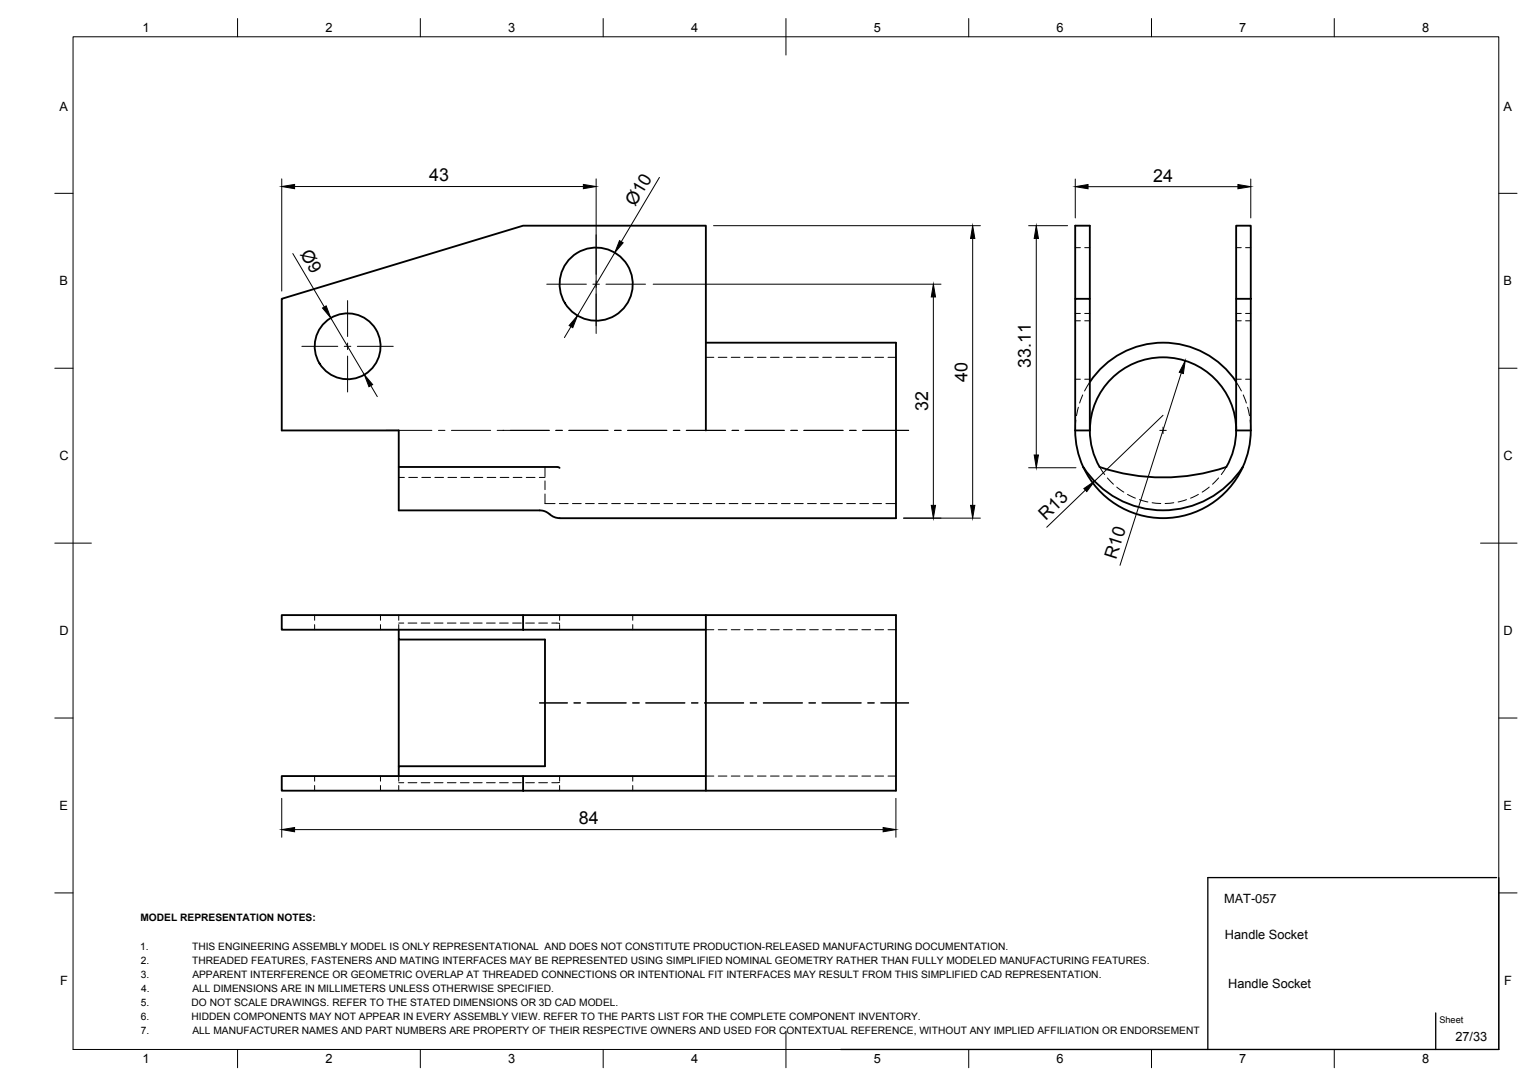
ISO-10303-21;
HEADER;
/* Generated by software containing ST-Developer
 * from STEP Tools, Inc. (www.steptools.com) 
 */

FILE_DESCRIPTION(
/* description */ ('STEP AP214', 'CAx-IF Rec.Pracs.---Representation and Presentation of Product Manufa
cturing Information (PMI)---4.0---2014-10-13'),
/* implementation_level */ '2;1');

FILE_NAME(
/* name */ 'Handle Socket.step',
/* time_stamp */ '2026-10-28T23:34:22+01:00',
/* author */ (''),
/* organization */ (''),
/* preprocessor_version */ 'ST-DEVELOPER v20.2',
/* originating_system */ 'Autodesk Translation Framework v15.17.0.0',
/* authorisation */ '');

FILE_SCHEMA (('AP242_MANAGED_MODEL_BASED_3D_ENGINEERING_MIM_LF { 1 0 10303 442 2 1 4 }'));
ENDSEC;

DATA;
#10=MECHANICAL_DESIGN_GEOMETRIC_PRESENTATION_REPRESENTATION('',(#268),#27807);
#220=SHAPE_REPRESENTATION_RELATIONSHIP('SRR','None',#27918,#242);
#242=ADVANCED_BREP_SHAPE_REPRESENTATION('',(#297),#27798);
#268=STYLED_ITEM('',(#28070),#297);
#297=MANIFOLD_SOLID_BREP('Body1',#12044);
#322=(
BOUNDED_SURFACE()
B_SPLINE_SURFACE(3,2,((#23001,#23002,#23003),(#23004,#23005,#23006),(#23007,
#23008,#23009),(#23010,#23011,#23012),(#23013,#23014,#23015),(#23016,#23017,
#23018),(#23019,#23020,#23021),(#23022,#23023,#23024),(#23025,#23026,#23027),
(#23028,#23029,#23030),(#23031,#23032,#23033),(#23034,#23035,#23036),(#23037,
#23038,#23039),(#23040,#23041,#23042),(#23043,#23044,#23045),(#23046,#23047,
#23048),(#23049,#23050,#23051),(#23052,#23053,#23054),(#23055,#23056,#23057),
(#23058,#23059,#23060),(#23061,#23062,#23063),(#23064,#23065,#23066),(#23067,
#23068,#23069),(#23070,#23071,#23072),(#23073,#23074,#23075),(#23076,#23077,
#23078),(#23079,#23080,#23081),(#23082,#23083,#23084),(#23085,#23086,#23087),
(#23088,#23089,#23090),(#23091,#23092,#23093),(#23094,#23095,#23096),(#23097,
#23098,#23099),(#23100,#23101,#23102),(#23103,#23104,#23105),(#23106,#23107,
#23108),(#23109,#23110,#23111),(#23112,#23113,#23114),(#23115,#23116,#23117),
(#23118,#23119,#23120),(#23121,#23122,#23123),(#23124,#23125,#23126),(#23127,
#23128,#23129),(#23130,#23131,#23132),(#23133,#23134,#23135),(#23136,#23137,
#23138),(#23139,#23140,#23141),(#23142,#23143,#23144),(#23145,#23146,#23147),
(#23148,#23149,#23150),(#23151,#23152,#23153),(#23154,#23155,#23156),(#23157,
#23158,#23159),(#23160,#23161,#23162)),.UNSPECIFIED.,.F.,.F.,.F.)
B_SPLINE_SURFACE_WITH_KNOTS((4,2,2,2,2,2,2,2,2,2,2,2,2,2,2,2,2,2,2,2,2,
2,2,2,2,2,4),(3,3),(0.0156830691858876,0.0164505202472942,0.0166981564596516,
0.0171934288843663,0.017688701309081,0.0181839737337957,0.0191745185832252,
0.0201650634326547,0.0221461531315136,0.0241272428303725,0.025117787679802,
0.0261083325292314,0.0280894222280904,0.0300705119269493,0.0320516016258082,
0.0360137810235261,0.037994870722385,0.0399759604212439,0.0419570501201028,
0.0439381398189618,0.0449286846683912,0.0459192295178207,0.0464145019425354,
0.0469097743672502,0.0474050467919649,0.0476526830043223,0.0484205987519554),
(-0.000176656774630185,1.00140559977643),.UNSPECIFIED.)
GEOMETRIC_REPRESENTATION_ITEM()
RATIONAL_B_SPLINE_SURFACE(((1.00000185229478,0.994749992386749,1.00001475620861),
(1.00000110311236,0.996873419742612,1.0000087878864),(1.00000061689249,
0.998251525466236,1.00000491444144),(1.00000073022143,0.99793031426867,
1.0000058172705),(1.00000081643938,0.997685944476427,1.00000650412124),
(1.00000116817153,0.996689020835744,1.00000930617684),(1.00000151293943,
0.995711836146633,1.00001205275212),(1.00000222875737,0.99368297460525,
1.00001775527797),(1.00000261226297,0.992595994639531,1.00002081045509),
(1.00000339798395,0.990369005078046,1.00002706985983),(1.00000379540439,
0.989242585902711,1.00003023588883),(1.00000499052043,0.985855237206275,
1.00003975671769),(1.00000579086045,0.983586812540499,1.00004613258417),
(1.00000737677408,0.97909181598218,1.00005876668146),(1.00000816422513,
0.976859922850868,1.00006503986867),(1.00001048220609,0.970290008684874,
1.0000835059417),(1.0000119461136,0.966140817279626,1.00009516808364),(1.00001468654717,
0.958373534637283,1.00011699960303),(1.00001596349836,0.954754238433,1.00012717236729),
(1.00001771880672,0.949779121960846,1.00014115593873),(1.00001827868632,
0.948192240535891,1.00014561619005),(1.00001932722233,0.945220347466773,
1.00015396929681),(1.00001981740926,0.943830997788028,1.00015787434518),
(1.00002118448659,0.939956254724288,1.00016876509453),(1.00002195823644,
0.937763195243397,1.00017492913191),(1.00002321565211,0.934199269074837,
1.00018494626748),(1.00002370061483,0.932824726524174,1.00018880969743),
(1.00002434501334,0.930998290964812,1.00019394326411),(1.00002450689124,
0.930539476192181,1.00019523285585),(1.00002450200607,0.930553322329606,
1.00019519393848),(1.00002385083742,0.932398946709429,1.00019000643775),
(1.00002196617021,0.937740708359039,1.00017499233585),(1.00002117811911,
0.939974302221974,1.00016871436838),(1.00001935011025,0.945155475621783,
1.00015415163226),(1.00001830824342,0.948108466066406,1.00014585165514),
(1.00001599049957,0.954677708176843,1.00012738747106),(1.0000147145338,
0.958294211383293,1.00011722255709),(1.00001194082592,0.966155804298885,
1.00009512595959),(1.00001046725737,0.97033237824493,1.00008338685348),
(1.00000815970583,0.976872732002048,1.00006500386596),(1.00000737308074,
0.979102284123733,1.00005873725863),(1.00000577774524,0.983623985306201,
1.0000460281026),(1.00000497387877,0.985902405097253,1.00003962414279),
(1.000003776533,0.989296073600137,1.00003008555083),(1.00000337746495,0.990427162612735,
1.00002690639631),(1.00000259754195,0.992637718792777,1.00002069318092),
(1.00000221666145,0.993717258376601,1.0000176589165),(1.00000150078254,
0.995746292719822,1.00001195590495),(1.00000115795301,0.996717983459339,
1.00000922477153),(1.00000081463085,0.997691070447167,1.00000648971367),
(1.00000072988353,0.997931272000135,1.0000058145786),(1.00000061781061,
0.99824892319208,1.00000492175566),(1.00000109047742,0.996909231281611,
1.00000868723083),(1.00000189977857,0.994615407843422,1.0000151344857)))
REPRESENTATION_ITEM('')
SURFACE()
);
#416=FACE_BOUND('',#2542,.T.);
#417=FACE_BOUND('',#2548,.T.);
#418=FACE_BOUND('',#2549,.T.);
#419=FACE_BOUND('',#2551,.T.);
#420=FACE_BOUND('',#2552,.T.);
#421=FACE_BOUND('',#2558,.T.);
#422=FACE_BOUND('',#2559,.T.);
#423=FACE_BOUND('',#2561,.T.);
#424=FACE_BOUND('',#2562,.T.);
#671=PLANE('',#13398);
#672=PLANE('',#13399);
#673=PLANE('',#13400);
#674=PLANE('',#13401);
#675=PLANE('',#13402);
#676=PLANE('',#13403);
#677=PLANE('',#13404);
#678=PLANE('',#13405);
#679=PLANE('',#13406);
#680=PLANE('',#13407);
#681=PLANE('',#13408);
#682=PLANE('',#13409);
#683=PLANE('',#13410);
#684=PLANE('',#13411);
#685=PLANE('',#13412);
#686=PLANE('',#13413);
#687=PLANE('',#13419);
#688=PLANE('',#13420);
#838=TOROIDAL_SURFACE('',#13421,10.,2.);
#920=B_SPLINE_CURVE_WITH_KNOTS('',3,(#22599,#22600,#22601,#22602,#22603,
#22604,#22605,#22606,#22607,#22608,#22609,#22610,#22611),.UNSPECIFIED.,
 .F.,.F.,(4,3,3,3,4),(-8.94491631300586E-6,0.000122293976412443,0.000196963243301103,
0.000348477111734026,0.000402871401407367),.UNSPECIFIED.);
#921=B_SPLINE_CURVE_WITH_KNOTS('',3,(#22635,#22636,#22637,#22638,#22639,
#22640,#22641,#22642,#22643,#22644,#22645,#22646,#22647),.UNSPECIFIED.,
 .F.,.F.,(4,3,3,3,4),(1.90501246655379E-12,0.000149886598358764,0.000203002185902805,
0.000344863019354018,0.000406004371347535),.UNSPECIFIED.);
#922=B_SPLINE_CURVE_WITH_KNOTS('',3,(#22716,#22717,#22718,#22719,#22720,
#22721,#22722,#22723,#22724,#22725,#22726,#22727,#22728,#22729,#22730,#22731,
#22732,#22733,#22734,#22735,#22736,#22737,#22738,#22739,#22740,#22741,#22742,
#22743,#22744,#22745,#22746,#22747,#22748,#22749,#22750,#22751,#22752,#22753,
#22754,#22755,#22756,#22757,#22758,#22759,#22760,#22761),.UNSPECIFIED.,
 .F.,.F.,(4,2,2,2,2,2,2,2,2,2,2,2,2,2,2,2,2,2,2,2,2,2,4),(0.,0.00042797836355374,
0.00085595672710748,0.00171191345421505,0.00256787018132261,0.00342382690843018,
0.00513574036264529,0.00684765381686041,0.00770361054396788,0.00855956727107535,
0.0102714807252903,0.0119833941795052,0.0136953076337201,0.0171191345421499,
0.0188310479963648,0.0205429614505798,0.0222548749047947,0.0239667883590096,
0.0248227450861171,0.0256787018132246,0.0265346585403321,0.0269626369038859,
0.0273906152674397),.UNSPECIFIED.);
#923=B_SPLINE_CURVE_WITH_KNOTS('',3,(#22766,#22767,#22768,#22769,#22770,
#22771,#22772,#22773,#22774,#22775,#22776,#22777,#22778,#22779,#22780,#22781,
#22782,#22783,#22784,#22785,#22786,#22787,#22788,#22789,#22790,#22791,#22792,
#22793,#22794,#22795,#22796,#22797,#22798,#22799,#22800,#22801,#22802,#22803,
#22804,#22805,#22806,#22807,#22808,#22809,#22810,#22811,#22812,#22813,#22814,
#22815,#22816,#22817,#22818,#22819,#22820,#22821,#22822,#22823,#22824,#22825,
#22826,#22827,#22828,#22829,#22830,#22831,#22832,#22833,#22834,#22835,#22836,
#22837,#22838,#22839,#22840,#22841,#22842,#22843,#22844,#22845,#22846,#22847,
#22848,#22849,#22850,#22851,#22852,#22853,#22854,#22855,#22856,#22857,#22858,
#22859,#22860,#22861,#22862,#22863,#22864,#22865,#22866,#22867,#22868,#22869,
#22870,#22871,#22872,#22873,#22874,#22875,#22876,#22877,#22878,#22879,#22880,
#22881,#22882,#22883,#22884,#22885,#22886,#22887,#22888,#22889,#22890,#22891,
#22892,#22893,#22894,#22895,#22896,#22897,#22898,#22899,#22900,#22901,#22902,
#22903,#22904,#22905,#22906,#22907,#22908,#22909,#22910,#22911,#22912,#22913,
#22914,#22915,#22916,#22917,#22918,#22919,#22920,#22921,#22922,#22923,#22924,
#22925,#22926,#22927,#22928,#22929,#22930,#22931,#22932,#22933,#22934,#22935,
#22936,#22937,#22938,#22939,#22940,#22941,#22942,#22943,#22944,#22945,#22946,
#22947,#22948,#22949,#22950,#22951,#22952,#22953,#22954,#22955,#22956,#22957,
#22958,#22959,#22960,#22961,#22962,#22963,#22964,#22965,#22966,#22967,#22968,
#22969,#22970,#22971,#22972,#22973,#22974,#22975,#22976,#22977,#22978,#22979,
#22980,#22981,#22982,#22983,#22984,#22985,#22986,#22987,#22988,#22989,#22990,
#22991,#22992,#22993,#22994,#22995,#22996,#22997,#22998,#22999,#23000),
 .UNSPECIFIED.,.F.,.F.,(4,3,3,3,3,3,3,3,3,3,3,3,3,3,3,3,3,3,3,3,3,3,3,3,
3,3,3,3,3,3,3,3,3,3,3,3,3,3,3,3,3,3,3,3,3,3,3,3,3,3,3,3,3,3,3,3,3,3,3,3,
3,3,3,3,3,3,3,3,3,3,3,3,3,3,3,3,3,3,4),(4.92899567643811E-13,6.25324094450888E-5,
0.000108135161089233,0.000169914174680728,0.000216270322178465,0.00030943720716885,
0.000413935938866143,0.000432540644356983,0.000574368182756462,0.000730585733412546,
0.000865081288713848,0.0011111676997501,0.00137115397560176,0.00165280502519303,
0.00173016257742746,0.0021631859889676,0.00262174667632143,0.00312444156864647,
0.00346032515485454,0.00399962729951328,0.00432540644356815,0.00475794708792495,
0.00519048773228175,0.00580087629302463,0.0064255985829778,0.00692065030970915,
0.00756964026772925,0.00822018102493731,0.00865081288713655,0.00908335353149343,
0.00949422462642801,0.00951589417585031,0.0101632105932538,0.0103809754645641,
0.0110451277363797,0.0117441709571396,0.0124097069791447,0.0130727965065704,
0.0137303575905069,0.0138413006194192,0.0145176167184007,0.0151956374788783,
0.0155714631968468,0.0160965814245652,0.0166216819946583,0.0171475979342611,
0.0173016257742743,0.0179650597324343,0.018627559129564,0.0190317883517019,
0.0198298746356556,0.0206344291379891,0.0207619509291294,0.0213868246193969,
0.022007159801814,0.022492113506557,0.0230625131047404,0.0236423945943625,
0.0241817119047142,0.0242222760839846,0.0246853332276435,0.0250873573726984,
0.0254771261541672,0.025844738861123,0.0259524386614121,0.0262218968916945,
0.0264777260220052,0.0267146153189825,0.0268175199501259,0.0269752262516356,
0.0271182846351551,0.0272500605944827,0.0273581957555719,0.0274515657429817,
0.0274663309166611,0.0275422189045734,0.0275744660777502,0.027633797106646,
0.0276826012383845),.UNSPECIFIED.);
#1167=CYLINDRICAL_SURFACE('',#13370,4.50000000000001);
#1168=CYLINDRICAL_SURFACE('',#13373,4.99999999999999);
#1169=CYLINDRICAL_SURFACE('',#13376,4.50000000000001);
#1170=CYLINDRICAL_SURFACE('',#13379,4.99999999999999);
#1171=CYLINDRICAL_SURFACE('',#13382,10.);
#1172=CYLINDRICAL_SURFACE('',#13389,12.);
#1173=CYLINDRICAL_SURFACE('',#13414,27.);
#1174=CYLINDRICAL_SURFACE('',#13417,13.);
#1754=FACE_OUTER_BOUND('',#2532,.T.);
#1755=FACE_OUTER_BOUND('',#2533,.T.);
#1756=FACE_OUTER_BOUND('',#2534,.T.);
#1757=FACE_OUTER_BOUND('',#2535,.T.);
#1758=FACE_OUTER_BOUND('',#2536,.T.);
#1759=FACE_OUTER_BOUND('',#2537,.T.);
#1760=FACE_OUTER_BOUND('',#2538,.T.);
#1761=FACE_OUTER_BOUND('',#2539,.T.);
#1762=FACE_OUTER_BOUND('',#2540,.T.);
#1763=FACE_OUTER_BOUND('',#2541,.T.);
#1764=FACE_OUTER_BOUND('',#2543,.T.);
#1765=FACE_OUTER_BOUND('',#2544,.T.);
#1766=FACE_OUTER_BOUND('',#2545,.T.);
#1767=FACE_OUTER_BOUND('',#2546,.T.);
#1768=FACE_OUTER_BOUND('',#2547,.T.);
#1769=FACE_OUTER_BOUND('',#2550,.T.);
#1770=FACE_OUTER_BOUND('',#2553,.T.);
#1771=FACE_OUTER_BOUND('',#2554,.T.);
#1772=FACE_OUTER_BOUND('',#2555,.T.);
#1773=FACE_OUTER_BOUND('',#2556,.T.);
#1774=FACE_OUTER_BOUND('',#2557,.T.);
#1775=FACE_OUTER_BOUND('',#2560,.T.);
#1776=FACE_OUTER_BOUND('',#2563,.T.);
#1777=FACE_OUTER_BOUND('',#2564,.T.);
#1778=FACE_OUTER_BOUND('',#2565,.T.);
#1779=FACE_OUTER_BOUND('',#2566,.T.);
#1780=FACE_OUTER_BOUND('',#2567,.T.);
#1781=FACE_OUTER_BOUND('',#2568,.T.);
#2532=EDGE_LOOP('',(#10371,#10372,#10373,#10374));
#2533=EDGE_LOOP('',(#10375,#10376,#10377,#10378));
#2534=EDGE_LOOP('',(#10379,#10380,#10381,#10382));
#2535=EDGE_LOOP('',(#10383,#10384,#10385,#10386));
#2536=EDGE_LOOP('',(#10387,#10388,#10389,#10390,#10391,#10392,#10393,#10394,
#10395,#10396,#10397,#10398));
#2537=EDGE_LOOP('',(#10399,#10400,#10401,#10402,#10403,#10404,#10405,#10406,
#10407,#10408,#10409,#10410,#10411,#10412,#10413,#10414));
#2538=EDGE_LOOP('',(#10415,#10416,#10417,#10418));
#2539=EDGE_LOOP('',(#10419,#10420,#10421,#10422));
#2540=EDGE_LOOP('',(#10423,#10424,#10425,#10426,#10427,#10428));
#2541=EDGE_LOOP('',(#10429));
#2542=EDGE_LOOP('',(#10430));
#2543=EDGE_LOOP('',(#10431,#10432,#10433,#10434));
#2544=EDGE_LOOP('',(#10435,#10436,#10437,#10438));
#2545=EDGE_LOOP('',(#10439,#10440,#10441,#10442));
#2546=EDGE_LOOP('',(#10443,#10444,#10445,#10446));
#2547=EDGE_LOOP('',(#10447,#10448,#10449,#10450,#10451,#10452));
#2548=EDGE_LOOP('',(#10453));
#2549=EDGE_LOOP('',(#10454));
#2550=EDGE_LOOP('',(#10455,#10456,#10457,#10458,#10459,#10460,#10461));
#2551=EDGE_LOOP('',(#10462));
#2552=EDGE_LOOP('',(#10463));
#2553=EDGE_LOOP('',(#10464,#10465,#10466,#10467));
#2554=EDGE_LOOP('',(#10468,#10469,#10470,#10471));
#2555=EDGE_LOOP('',(#10472,#10473,#10474,#10475));
#2556=EDGE_LOOP('',(#10476,#10477,#10478,#10479));
#2557=EDGE_LOOP('',(#10480,#10481,#10482,#10483,#10484,#10485));
#2558=EDGE_LOOP('',(#10486));
#2559=EDGE_LOOP('',(#10487));
#2560=EDGE_LOOP('',(#10488,#10489,#10490,#10491,#10492,#10493,#10494));
#2561=EDGE_LOOP('',(#10495));
#2562=EDGE_LOOP('',(#10496));
#2563=EDGE_LOOP('',(#10497,#10498,#10499,#10500));
#2564=EDGE_LOOP('',(#10501,#10502,#10503,#10504));
#2565=EDGE_LOOP('',(#10505,#10506,#10507,#10508,#10509,#10510,#10511,#10512));
#2566=EDGE_LOOP('',(#10513,#10514));
#2567=EDGE_LOOP('',(#10515,#10516));
#2568=EDGE_LOOP('',(#10517,#10518,#10519,#10520));
#3372=LINE('',#22552,#4192);
#3373=LINE('',#22558,#4193);
#3374=LINE('',#22564,#4194);
#3375=LINE('',#22570,#4195);
#3376=LINE('',#22576,#4196);
#3377=LINE('',#22580,#4197);
#3378=LINE('',#22584,#4198);
#3379=LINE('',#22588,#4199);
#3380=LINE('',#22592,#4200);
#3381=LINE('',#22613,#4201);
#3382=LINE('',#22617,#4202);
#3383=LINE('',#22623,#4203);
#3384=LINE('',#22630,#4204);
#3385=LINE('',#22634,#4205);
#3386=LINE('',#22650,#4206);
#3387=LINE('',#22651,#4207);
#3388=LINE('',#22653,#4208);
#3389=LINE('',#22654,#4209);
#3390=LINE('',#22656,#4210);
#3391=LINE('',#22658,#4211);
#3392=LINE('',#22660,#4212);
#3393=LINE('',#22661,#4213);
#3394=LINE('',#22663,#4214);
#3395=LINE('',#22664,#4215);
#3396=LINE('',#22668,#4216);
#3397=LINE('',#22670,#4217);
#3398=LINE('',#22671,#4218);
#3399=LINE('',#22674,#4219);
#3400=LINE('',#22676,#4220);
#3401=LINE('',#22677,#4221);
#3402=LINE('',#22680,#4222);
#3403=LINE('',#22682,#4223);
#3404=LINE('',#22683,#4224);
#3405=LINE('',#22685,#4225);
#3406=LINE('',#22686,#4226);
#3407=LINE('',#22691,#4227);
#3408=LINE('',#22693,#4228);
#3409=LINE('',#22694,#4229);
#3410=LINE('',#22697,#4230);
#3411=LINE('',#22699,#4231);
#3412=LINE('',#22700,#4232);
#3413=LINE('',#22703,#4233);
#3414=LINE('',#22705,#4234);
#3415=LINE('',#22706,#4235);
#3416=LINE('',#22708,#4236);
#3417=LINE('',#22709,#4237);
#4192=VECTOR('',#16498,4.50000000000001);
#4193=VECTOR('',#16505,4.99999999999999);
#4194=VECTOR('',#16512,4.50000000000001);
#4195=VECTOR('',#16519,4.99999999999999);
#4196=VECTOR('',#16526,10.);
#4197=VECTOR('',#16529,1000.);
#4198=VECTOR('',#16532,1000.);
#4199=VECTOR('',#16535,1000.);
#4200=VECTOR('',#16538,1000.);
#4201=VECTOR('',#16545,1000.);
#4202=VECTOR('',#16548,1000.);
#4203=VECTOR('',#16553,12.);
#4204=VECTOR('',#16560,1000.);
#4205=VECTOR('',#16563,1000.);
#4206=VECTOR('',#16566,1000.);
#4207=VECTOR('',#16567,1000.);
#4208=VECTOR('',#16568,1000.);
#4209=VECTOR('',#16569,1000.);
#4210=VECTOR('',#16572,1000.);
#4211=VECTOR('',#16573,1000.);
#4212=VECTOR('',#16574,1000.);
#4213=VECTOR('',#16575,1000.);
#4214=VECTOR('',#16578,1000.);
#4215=VECTOR('',#16579,1000.);
#4216=VECTOR('',#16584,1000.);
#4217=VECTOR('',#16585,1000.);
#4218=VECTOR('',#16586,1000.);
#4219=VECTOR('',#16589,1000.);
#4220=VECTOR('',#16590,1000.);
#4221=VECTOR('',#16591,1000.);
#4222=VECTOR('',#16594,1000.);
#4223=VECTOR('',#16595,1000.);
#4224=VECTOR('',#16596,1000.);
#4225=VECTOR('',#16599,1000.);
#4226=VECTOR('',#16600,1000.);
#4227=VECTOR('',#16607,1000.);
#4228=VECTOR('',#16608,1000.);
#4229=VECTOR('',#16609,1000.);
#4230=VECTOR('',#16612,1000.);
#4231=VECTOR('',#16613,1000.);
#4232=VECTOR('',#16614,1000.);
#4233=VECTOR('',#16617,1000.);
#4234=VECTOR('',#16618,1000.);
#4235=VECTOR('',#16619,1000.);
#4236=VECTOR('',#16622,1000.);
#4237=VECTOR('',#16623,1000.);
#4893=CIRCLE('',#13371,4.50000000000001);
#4894=CIRCLE('',#13372,4.50000000000001);
#4895=CIRCLE('',#13374,4.99999999999999);
#4896=CIRCLE('',#13375,4.99999999999999);
#4897=CIRCLE('',#13377,4.50000000000001);
#4898=CIRCLE('',#13378,4.50000000000001);
#4899=CIRCLE('',#13380,4.99999999999999);
#4900=CIRCLE('',#13381,4.99999999999999);
#4901=CIRCLE('',#13383,10.);
#4902=CIRCLE('',#13384,10.);
#4903=CIRCLE('',#13385,10.);
#4904=CIRCLE('',#13386,10.);
#4905=CIRCLE('',#13387,10.);
#4906=CIRCLE('',#13388,10.);
#4907=CIRCLE('',#13390,12.);
#4908=CIRCLE('',#13391,12.);
#4909=CIRCLE('',#13392,12.);
#4910=CIRCLE('',#13393,12.);
#4911=CIRCLE('',#13394,12.);
#4912=CIRCLE('',#13395,12.);
#4913=CIRCLE('',#13396,12.);
#4914=CIRCLE('',#13397,12.);
#4915=CIRCLE('',#13415,27.);
#4916=CIRCLE('',#13416,27.);
#4917=CIRCLE('',#13418,13.);
#5843=VERTEX_POINT('',#22549);
#5844=VERTEX_POINT('',#22551);
#5845=VERTEX_POINT('',#22555);
#5846=VERTEX_POINT('',#22557);
#5847=VERTEX_POINT('',#22561);
#5848=VERTEX_POINT('',#22563);
#5849=VERTEX_POINT('',#22567);
#5850=VERTEX_POINT('',#22569);
#5851=VERTEX_POINT('',#22573);
#5852=VERTEX_POINT('',#22575);
#5853=VERTEX_POINT('',#22577);
#5854=VERTEX_POINT('',#22579);
#5855=VERTEX_POINT('',#22581);
#5856=VERTEX_POINT('',#22583);
#5857=VERTEX_POINT('',#22585);
#5858=VERTEX_POINT('',#22587);
#5859=VERTEX_POINT('',#22589);
#5860=VERTEX_POINT('',#22591);
#5861=VERTEX_POINT('',#22595);
#5862=VERTEX_POINT('',#22596);
#5863=VERTEX_POINT('',#22598);
#5864=VERTEX_POINT('',#22612);
#5865=VERTEX_POINT('',#22614);
#5866=VERTEX_POINT('',#22616);
#5867=VERTEX_POINT('',#22618);
#5868=VERTEX_POINT('',#22620);
#5869=VERTEX_POINT('',#22622);
#5870=VERTEX_POINT('',#22625);
#5871=VERTEX_POINT('',#22627);
#5872=VERTEX_POINT('',#22629);
#5873=VERTEX_POINT('',#22631);
#5874=VERTEX_POINT('',#22633);
#5875=VERTEX_POINT('',#22649);
#5876=VERTEX_POINT('',#22652);
#5877=VERTEX_POINT('',#22657);
#5878=VERTEX_POINT('',#22659);
#5879=VERTEX_POINT('',#22667);
#5880=VERTEX_POINT('',#22669);
#5881=VERTEX_POINT('',#22673);
#5882=VERTEX_POINT('',#22675);
#5883=VERTEX_POINT('',#22679);
#5884=VERTEX_POINT('',#22681);
#5885=VERTEX_POINT('',#22690);
#5886=VERTEX_POINT('',#22692);
#5887=VERTEX_POINT('',#22696);
#5888=VERTEX_POINT('',#22698);
#5889=VERTEX_POINT('',#22702);
#5890=VERTEX_POINT('',#22704);
#7398=EDGE_CURVE('',#5843,#5843,#4893,.T.);
#7399=EDGE_CURVE('',#5843,#5844,#3372,.T.);
#7400=EDGE_CURVE('',#5844,#5844,#4894,.T.);
#7401=EDGE_CURVE('',#5845,#5845,#4895,.T.);
#7402=EDGE_CURVE('',#5845,#5846,#3373,.T.);
#7403=EDGE_CURVE('',#5846,#5846,#4896,.T.);
#7404=EDGE_CURVE('',#5847,#5847,#4897,.T.);
#7405=EDGE_CURVE('',#5847,#5848,#3374,.T.);
#7406=EDGE_CURVE('',#5848,#5848,#4898,.T.);
#7407=EDGE_CURVE('',#5849,#5849,#4899,.T.);
#7408=EDGE_CURVE('',#5849,#5850,#3375,.T.);
#7409=EDGE_CURVE('',#5850,#5850,#4900,.T.);
#7410=EDGE_CURVE('',#5851,#5851,#4901,.T.);
#7411=EDGE_CURVE('',#5851,#5852,#3376,.T.);
#7412=EDGE_CURVE('',#5852,#5853,#4902,.T.);
#7413=EDGE_CURVE('',#5854,#5853,#3377,.T.);
#7414=EDGE_CURVE('',#5855,#5854,#4903,.T.);
#7415=EDGE_CURVE('',#5855,#5856,#3378,.T.);
#7416=EDGE_CURVE('',#5857,#5856,#4904,.T.);
#7417=EDGE_CURVE('',#5858,#5857,#3379,.T.);
#7418=EDGE_CURVE('',#5859,#5858,#4905,.T.);
#7419=EDGE_CURVE('',#5860,#5859,#3380,.T.);
#7420=EDGE_CURVE('',#5860,#5852,#4906,.T.);
#7421=EDGE_CURVE('',#5861,#5862,#4907,.T.);
#7422=EDGE_CURVE('',#5862,#5863,#920,.T.);
#7423=EDGE_CURVE('',#5864,#5863,#3381,.T.);
#7424=EDGE_CURVE('',#5865,#5864,#4908,.T.);
#7425=EDGE_CURVE('',#5865,#5866,#3382,.T.);
#7426=EDGE_CURVE('',#5866,#5867,#4909,.T.);
#7427=EDGE_CURVE('',#5868,#5867,#4910,.T.);
#7428=EDGE_CURVE('',#5868,#5869,#3383,.T.);
#7429=EDGE_CURVE('',#5869,#5869,#4911,.T.);
#7430=EDGE_CURVE('',#5870,#5868,#4912,.T.);
#7431=EDGE_CURVE('',#5871,#5870,#4913,.T.);
#7432=EDGE_CURVE('',#5871,#5872,#3384,.T.);
#7433=EDGE_CURVE('',#5873,#5872,#4914,.T.);
#7434=EDGE_CURVE('',#5873,#5874,#3385,.T.);
#7435=EDGE_CURVE('',#5874,#5861,#921,.T.);
#7436=EDGE_CURVE('',#5859,#5875,#3386,.T.);
#7437=EDGE_CURVE('',#5872,#5859,#3387,.T.);
#7438=EDGE_CURVE('',#5872,#5876,#3388,.T.);
#7439=EDGE_CURVE('',#5876,#5875,#3389,.T.);
#7440=EDGE_CURVE('',#5854,#5865,#3390,.T.);
#7441=EDGE_CURVE('',#5854,#5877,#3391,.T.);
#7442=EDGE_CURVE('',#5878,#5877,#3392,.T.);
#7443=EDGE_CURVE('',#5865,#5878,#3393,.T.);
#7444=EDGE_CURVE('',#5853,#5867,#3394,.T.);
#7445=EDGE_CURVE('',#5860,#5870,#3395,.T.);
#7446=EDGE_CURVE('',#5871,#5879,#3396,.T.);
#7447=EDGE_CURVE('',#5870,#5880,#3397,.T.);
#7448=EDGE_CURVE('',#5879,#5880,#3398,.T.);
#7449=EDGE_CURVE('',#5880,#5881,#3399,.T.);
#7450=EDGE_CURVE('',#5882,#5881,#3400,.T.);
#7451=EDGE_CURVE('',#5879,#5882,#3401,.T.);
#7452=EDGE_CURVE('',#5881,#5883,#3402,.T.);
#7453=EDGE_CURVE('',#5884,#5883,#3403,.T.);
#7454=EDGE_CURVE('',#5882,#5884,#3404,.T.);
#7455=EDGE_CURVE('',#5875,#5883,#3405,.T.);
#7456=EDGE_CURVE('',#5876,#5884,#3406,.T.);
#7457=EDGE_CURVE('',#5866,#5885,#3407,.T.);
#7458=EDGE_CURVE('',#5885,#5886,#3408,.T.);
#7459=EDGE_CURVE('',#5867,#5886,#3409,.T.);
#7460=EDGE_CURVE('',#5886,#5887,#3410,.T.);
#7461=EDGE_CURVE('',#5885,#5888,#3411,.T.);
#7462=EDGE_CURVE('',#5888,#5887,#3412,.T.);
#7463=EDGE_CURVE('',#5877,#5889,#3413,.T.);
#7464=EDGE_CURVE('',#5890,#5889,#3414,.T.);
#7465=EDGE_CURVE('',#5878,#5890,#3415,.T.);
#7466=EDGE_CURVE('',#5887,#5889,#3416,.T.);
#7467=EDGE_CURVE('',#5888,#5890,#3417,.T.);
#7468=EDGE_CURVE('',#5857,#5856,#4915,.T.);
#7469=EDGE_CURVE('',#5858,#5855,#4916,.T.);
#7470=EDGE_CURVE('',#5863,#5874,#922,.T.);
#7471=EDGE_CURVE('',#5864,#5873,#4917,.T.);
#7472=EDGE_CURVE('',#5861,#5862,#923,.T.);
#10371=ORIENTED_EDGE('',*,*,#7398,.F.);
#10372=ORIENTED_EDGE('',*,*,#7399,.T.);
#10373=ORIENTED_EDGE('',*,*,#7400,.T.);
#10374=ORIENTED_EDGE('',*,*,#7399,.F.);
#10375=ORIENTED_EDGE('',*,*,#7401,.F.);
#10376=ORIENTED_EDGE('',*,*,#7402,.T.);
#10377=ORIENTED_EDGE('',*,*,#7403,.T.);
#10378=ORIENTED_EDGE('',*,*,#7402,.F.);
#10379=ORIENTED_EDGE('',*,*,#7404,.T.);
#10380=ORIENTED_EDGE('',*,*,#7405,.T.);
#10381=ORIENTED_EDGE('',*,*,#7406,.F.);
#10382=ORIENTED_EDGE('',*,*,#7405,.F.);
#10383=ORIENTED_EDGE('',*,*,#7407,.T.);
#10384=ORIENTED_EDGE('',*,*,#7408,.T.);
#10385=ORIENTED_EDGE('',*,*,#7409,.F.);
#10386=ORIENTED_EDGE('',*,*,#7408,.F.);
#10387=ORIENTED_EDGE('',*,*,#7410,.T.);
#10388=ORIENTED_EDGE('',*,*,#7411,.T.);
#10389=ORIENTED_EDGE('',*,*,#7412,.T.);
#10390=ORIENTED_EDGE('',*,*,#7413,.F.);
#10391=ORIENTED_EDGE('',*,*,#7414,.F.);
#10392=ORIENTED_EDGE('',*,*,#7415,.T.);
#10393=ORIENTED_EDGE('',*,*,#7416,.F.);
#10394=ORIENTED_EDGE('',*,*,#7417,.F.);
#10395=ORIENTED_EDGE('',*,*,#7418,.F.);
#10396=ORIENTED_EDGE('',*,*,#7419,.F.);
#10397=ORIENTED_EDGE('',*,*,#7420,.T.);
#10398=ORIENTED_EDGE('',*,*,#7411,.F.);
#10399=ORIENTED_EDGE('',*,*,#7421,.T.);
#10400=ORIENTED_EDGE('',*,*,#7422,.T.);
#10401=ORIENTED_EDGE('',*,*,#7423,.F.);
#10402=ORIENTED_EDGE('',*,*,#7424,.F.);
#10403=ORIENTED_EDGE('',*,*,#7425,.T.);
#10404=ORIENTED_EDGE('',*,*,#7426,.T.);
#10405=ORIENTED_EDGE('',*,*,#7427,.F.);
#10406=ORIENTED_EDGE('',*,*,#7428,.T.);
#10407=ORIENTED_EDGE('',*,*,#7429,.F.);
#10408=ORIENTED_EDGE('',*,*,#7428,.F.);
#10409=ORIENTED_EDGE('',*,*,#7430,.F.);
#10410=ORIENTED_EDGE('',*,*,#7431,.F.);
#10411=ORIENTED_EDGE('',*,*,#7432,.T.);
#10412=ORIENTED_EDGE('',*,*,#7433,.F.);
#10413=ORIENTED_EDGE('',*,*,#7434,.T.);
#10414=ORIENTED_EDGE('',*,*,#7435,.T.);
#10415=ORIENTED_EDGE('',*,*,#7436,.F.);
#10416=ORIENTED_EDGE('',*,*,#7437,.F.);
#10417=ORIENTED_EDGE('',*,*,#7438,.T.);
#10418=ORIENTED_EDGE('',*,*,#7439,.T.);
#10419=ORIENTED_EDGE('',*,*,#7440,.F.);
#10420=ORIENTED_EDGE('',*,*,#7441,.T.);
#10421=ORIENTED_EDGE('',*,*,#7442,.F.);
#10422=ORIENTED_EDGE('',*,*,#7443,.F.);
#10423=ORIENTED_EDGE('',*,*,#7430,.T.);
#10424=ORIENTED_EDGE('',*,*,#7427,.T.);
#10425=ORIENTED_EDGE('',*,*,#7444,.F.);
#10426=ORIENTED_EDGE('',*,*,#7412,.F.);
#10427=ORIENTED_EDGE('',*,*,#7420,.F.);
#10428=ORIENTED_EDGE('',*,*,#7445,.T.);
#10429=ORIENTED_EDGE('',*,*,#7429,.T.);
#10430=ORIENTED_EDGE('',*,*,#7410,.F.);
#10431=ORIENTED_EDGE('',*,*,#7446,.F.);
#10432=ORIENTED_EDGE('',*,*,#7431,.T.);
#10433=ORIENTED_EDGE('',*,*,#7447,.T.);
#10434=ORIENTED_EDGE('',*,*,#7448,.F.);
#10435=ORIENTED_EDGE('',*,*,#7449,.T.);
#10436=ORIENTED_EDGE('',*,*,#7450,.F.);
#10437=ORIENTED_EDGE('',*,*,#7451,.F.);
#10438=ORIENTED_EDGE('',*,*,#7448,.T.);
#10439=ORIENTED_EDGE('',*,*,#7452,.T.);
#10440=ORIENTED_EDGE('',*,*,#7453,.F.);
#10441=ORIENTED_EDGE('',*,*,#7454,.F.);
#10442=ORIENTED_EDGE('',*,*,#7450,.T.);
#10443=ORIENTED_EDGE('',*,*,#7455,.F.);
#10444=ORIENTED_EDGE('',*,*,#7439,.F.);
#10445=ORIENTED_EDGE('',*,*,#7456,.T.);
#10446=ORIENTED_EDGE('',*,*,#7453,.T.);
#10447=ORIENTED_EDGE('',*,*,#7451,.T.);
#10448=ORIENTED_EDGE('',*,*,#7454,.T.);
#10449=ORIENTED_EDGE('',*,*,#7456,.F.);
#10450=ORIENTED_EDGE('',*,*,#7438,.F.);
#10451=ORIENTED_EDGE('',*,*,#7432,.F.);
#10452=ORIENTED_EDGE('',*,*,#7446,.T.);
#10453=ORIENTED_EDGE('',*,*,#7404,.F.);
#10454=ORIENTED_EDGE('',*,*,#7407,.F.);
#10455=ORIENTED_EDGE('',*,*,#7449,.F.);
#10456=ORIENTED_EDGE('',*,*,#7447,.F.);
#10457=ORIENTED_EDGE('',*,*,#7445,.F.);
#10458=ORIENTED_EDGE('',*,*,#7419,.T.);
#10459=ORIENTED_EDGE('',*,*,#7436,.T.);
#10460=ORIENTED_EDGE('',*,*,#7455,.T.);
#10461=ORIENTED_EDGE('',*,*,#7452,.F.);
#10462=ORIENTED_EDGE('',*,*,#7406,.T.);
#10463=ORIENTED_EDGE('',*,*,#7409,.T.);
#10464=ORIENTED_EDGE('',*,*,#7426,.F.);
#10465=ORIENTED_EDGE('',*,*,#7457,.T.);
#10466=ORIENTED_EDGE('',*,*,#7458,.T.);
#10467=ORIENTED_EDGE('',*,*,#7459,.F.);
#10468=ORIENTED_EDGE('',*,*,#7460,.F.);
#10469=ORIENTED_EDGE('',*,*,#7458,.F.);
#10470=ORIENTED_EDGE('',*,*,#7461,.T.);
#10471=ORIENTED_EDGE('',*,*,#7462,.T.);
#10472=ORIENTED_EDGE('',*,*,#7463,.T.);
#10473=ORIENTED_EDGE('',*,*,#7464,.F.);
#10474=ORIENTED_EDGE('',*,*,#7465,.F.);
#10475=ORIENTED_EDGE('',*,*,#7442,.T.);
#10476=ORIENTED_EDGE('',*,*,#7466,.F.);
#10477=ORIENTED_EDGE('',*,*,#7462,.F.);
#10478=ORIENTED_EDGE('',*,*,#7467,.T.);
#10479=ORIENTED_EDGE('',*,*,#7464,.T.);
#10480=ORIENTED_EDGE('',*,*,#7461,.F.);
#10481=ORIENTED_EDGE('',*,*,#7457,.F.);
#10482=ORIENTED_EDGE('',*,*,#7425,.F.);
#10483=ORIENTED_EDGE('',*,*,#7443,.T.);
#10484=ORIENTED_EDGE('',*,*,#7465,.T.);
#10485=ORIENTED_EDGE('',*,*,#7467,.F.);
#10486=ORIENTED_EDGE('',*,*,#7398,.T.);
#10487=ORIENTED_EDGE('',*,*,#7401,.T.);
#10488=ORIENTED_EDGE('',*,*,#7460,.T.);
#10489=ORIENTED_EDGE('',*,*,#7466,.T.);
#10490=ORIENTED_EDGE('',*,*,#7463,.F.);
#10491=ORIENTED_EDGE('',*,*,#7441,.F.);
#10492=ORIENTED_EDGE('',*,*,#7413,.T.);
#10493=ORIENTED_EDGE('',*,*,#7444,.T.);
#10494=ORIENTED_EDGE('',*,*,#7459,.T.);
#10495=ORIENTED_EDGE('',*,*,#7400,.F.);
#10496=ORIENTED_EDGE('',*,*,#7403,.F.);
#10497=ORIENTED_EDGE('',*,*,#7468,.T.);
#10498=ORIENTED_EDGE('',*,*,#7415,.F.);
#10499=ORIENTED_EDGE('',*,*,#7469,.F.);
#10500=ORIENTED_EDGE('',*,*,#7417,.T.);
#10501=ORIENTED_EDGE('',*,*,#7423,.T.);
#10502=ORIENTED_EDGE('',*,*,#7470,.T.);
#10503=ORIENTED_EDGE('',*,*,#7434,.F.);
#10504=ORIENTED_EDGE('',*,*,#7471,.F.);
#10505=ORIENTED_EDGE('',*,*,#7418,.T.);
#10506=ORIENTED_EDGE('',*,*,#7469,.T.);
#10507=ORIENTED_EDGE('',*,*,#7414,.T.);
#10508=ORIENTED_EDGE('',*,*,#7440,.T.);
#10509=ORIENTED_EDGE('',*,*,#7424,.T.);
#10510=ORIENTED_EDGE('',*,*,#7471,.T.);
#10511=ORIENTED_EDGE('',*,*,#7433,.T.);
#10512=ORIENTED_EDGE('',*,*,#7437,.T.);
#10513=ORIENTED_EDGE('',*,*,#7468,.F.);
#10514=ORIENTED_EDGE('',*,*,#7416,.T.);
#10515=ORIENTED_EDGE('',*,*,#7421,.F.);
#10516=ORIENTED_EDGE('',*,*,#7472,.T.);
#10517=ORIENTED_EDGE('',*,*,#7422,.F.);
#10518=ORIENTED_EDGE('',*,*,#7472,.F.);
#10519=ORIENTED_EDGE('',*,*,#7435,.F.);
#10520=ORIENTED_EDGE('',*,*,#7470,.F.);
#11836=ADVANCED_FACE('',(#1754),#1167,.F.);
#11837=ADVANCED_FACE('',(#1755),#1168,.F.);
#11838=ADVANCED_FACE('',(#1756),#1169,.F.);
#11839=ADVANCED_FACE('',(#1757),#1170,.F.);
#11840=ADVANCED_FACE('',(#1758),#1171,.F.);
#11841=ADVANCED_FACE('',(#1759),#1172,.T.);
#11842=ADVANCED_FACE('',(#1760),#671,.T.);
#11843=ADVANCED_FACE('',(#1761),#672,.F.);
#11844=ADVANCED_FACE('',(#1762),#673,.T.);
#11845=ADVANCED_FACE('',(#1763,#416),#674,.T.);
#11846=ADVANCED_FACE('',(#1764),#675,.F.);
#11847=ADVANCED_FACE('',(#1765),#676,.F.);
#11848=ADVANCED_FACE('',(#1766),#677,.F.);
#11849=ADVANCED_FACE('',(#1767),#678,.T.);
#11850=ADVANCED_FACE('',(#1768,#417,#418),#679,.T.);
#11851=ADVANCED_FACE('',(#1769,#419,#420),#680,.F.);
#11852=ADVANCED_FACE('',(#1770),#681,.T.);
#11853=ADVANCED_FACE('',(#1771),#682,.T.);
#11854=ADVANCED_FACE('',(#1772),#683,.F.);
#11855=ADVANCED_FACE('',(#1773),#684,.T.);
#11856=ADVANCED_FACE('',(#1774,#421,#422),#685,.T.);
#11857=ADVANCED_FACE('',(#1775,#423,#424),#686,.F.);
#11858=ADVANCED_FACE('',(#1776),#1173,.F.);
#11859=ADVANCED_FACE('',(#1777),#1174,.T.);
#11860=ADVANCED_FACE('',(#1778),#687,.F.);
#11861=ADVANCED_FACE('',(#1779),#688,.T.);
#11862=ADVANCED_FACE('',(#1780),#838,.T.);
#11863=ADVANCED_FACE('',(#1781),#322,.F.);
#12044=CLOSED_SHELL('',(#11836,#11837,#11838,#11839,#11840,#11841,#11842,
#11843,#11844,#11845,#11846,#11847,#11848,#11849,#11850,#11851,#11852,#11853,
#11854,#11855,#11856,#11857,#11858,#11859,#11860,#11861,#11862,#11863));
#13369=AXIS2_PLACEMENT_3D('',#22547,#16492,#16493);
#13370=AXIS2_PLACEMENT_3D('',#22548,#16494,#16495);
#13371=AXIS2_PLACEMENT_3D('',#22550,#16496,#16497);
#13372=AXIS2_PLACEMENT_3D('',#22553,#16499,#16500);
#13373=AXIS2_PLACEMENT_3D('',#22554,#16501,#16502);
#13374=AXIS2_PLACEMENT_3D('',#22556,#16503,#16504);
#13375=AXIS2_PLACEMENT_3D('',#22559,#16506,#16507);
#13376=AXIS2_PLACEMENT_3D('',#22560,#16508,#16509);
#13377=AXIS2_PLACEMENT_3D('',#22562,#16510,#16511);
#13378=AXIS2_PLACEMENT_3D('',#22565,#16513,#16514);
#13379=AXIS2_PLACEMENT_3D('',#22566,#16515,#16516);
#13380=AXIS2_PLACEMENT_3D('',#22568,#16517,#16518);
#13381=AXIS2_PLACEMENT_3D('',#22571,#16520,#16521);
#13382=AXIS2_PLACEMENT_3D('',#22572,#16522,#16523);
#13383=AXIS2_PLACEMENT_3D('',#22574,#16524,#16525);
#13384=AXIS2_PLACEMENT_3D('',#22578,#16527,#16528);
#13385=AXIS2_PLACEMENT_3D('',#22582,#16530,#16531);
#13386=AXIS2_PLACEMENT_3D('',#22586,#16533,#16534);
#13387=AXIS2_PLACEMENT_3D('',#22590,#16536,#16537);
#13388=AXIS2_PLACEMENT_3D('',#22593,#16539,#16540);
#13389=AXIS2_PLACEMENT_3D('',#22594,#16541,#16542);
#13390=AXIS2_PLACEMENT_3D('',#22597,#16543,#16544);
#13391=AXIS2_PLACEMENT_3D('',#22615,#16546,#16547);
#13392=AXIS2_PLACEMENT_3D('',#22619,#16549,#16550);
#13393=AXIS2_PLACEMENT_3D('',#22621,#16551,#16552);
#13394=AXIS2_PLACEMENT_3D('',#22624,#16554,#16555);
#13395=AXIS2_PLACEMENT_3D('',#22626,#16556,#16557);
#13396=AXIS2_PLACEMENT_3D('',#22628,#16558,#16559);
#13397=AXIS2_PLACEMENT_3D('',#22632,#16561,#16562);
#13398=AXIS2_PLACEMENT_3D('',#22648,#16564,#16565);
#13399=AXIS2_PLACEMENT_3D('',#22655,#16570,#16571);
#13400=AXIS2_PLACEMENT_3D('',#22662,#16576,#16577);
#13401=AXIS2_PLACEMENT_3D('',#22665,#16580,#16581);
#13402=AXIS2_PLACEMENT_3D('',#22666,#16582,#16583);
#13403=AXIS2_PLACEMENT_3D('',#22672,#16587,#16588);
#13404=AXIS2_PLACEMENT_3D('',#22678,#16592,#16593);
#13405=AXIS2_PLACEMENT_3D('',#22684,#16597,#16598);
#13406=AXIS2_PLACEMENT_3D('',#22687,#16601,#16602);
#13407=AXIS2_PLACEMENT_3D('',#22688,#16603,#16604);
#13408=AXIS2_PLACEMENT_3D('',#22689,#16605,#16606);
#13409=AXIS2_PLACEMENT_3D('',#22695,#16610,#16611);
#13410=AXIS2_PLACEMENT_3D('',#22701,#16615,#16616);
#13411=AXIS2_PLACEMENT_3D('',#22707,#16620,#16621);
#13412=AXIS2_PLACEMENT_3D('',#22710,#16624,#16625);
#13413=AXIS2_PLACEMENT_3D('',#22711,#16626,#16627);
#13414=AXIS2_PLACEMENT_3D('',#22712,#16628,#16629);
#13415=AXIS2_PLACEMENT_3D('',#22713,#16630,#16631);
#13416=AXIS2_PLACEMENT_3D('',#22714,#16632,#16633);
#13417=AXIS2_PLACEMENT_3D('',#22715,#16634,#16635);
#13418=AXIS2_PLACEMENT_3D('',#22762,#16636,#16637);
#13419=AXIS2_PLACEMENT_3D('',#22763,#16638,#16639);
#13420=AXIS2_PLACEMENT_3D('',#22764,#16640,#16641);
#13421=AXIS2_PLACEMENT_3D('',#22765,#16642,#16643);
#16492=DIRECTION('axis',(0.,0.,1.));
#16493=DIRECTION('refdir',(1.,0.,0.));
#16494=DIRECTION('center_axis',(-2.73022310513781E-17,4.45132926068947E-17,
-1.));
#16495=DIRECTION('ref_axis',(0.852431871234064,0.522838316216775,-3.69481375527776E-23));
#16496=DIRECTION('center_axis',(-2.73022310513781E-17,4.45132926068947E-17,
-1.));
#16497=DIRECTION('ref_axis',(0.852431871234064,0.522838316216775,-3.69481375527776E-23));
#16498=DIRECTION('',(-2.73022310513781E-17,4.45132926068947E-17,-1.));
#16499=DIRECTION('center_axis',(-2.73022310513781E-17,4.45132926068947E-17,
-1.));
#16500=DIRECTION('ref_axis',(0.852431871234064,0.522838316216775,-3.69481375527776E-23));
#16501=DIRECTION('center_axis',(-2.73022310513781E-17,4.45132926068947E-17,
-1.));
#16502=DIRECTION('ref_axis',(0.852431871234061,0.522838316216779,-3.69481373062586E-23));
#16503=DIRECTION('center_axis',(-2.73022310513781E-17,4.45132926068947E-17,
-1.));
#16504=DIRECTION('ref_axis',(0.852431871234061,0.522838316216779,-3.69481373062586E-23));
#16505=DIRECTION('',(-2.73022310513781E-17,4.45132926068947E-17,-1.));
#16506=DIRECTION('center_axis',(-2.73022310513781E-17,4.45132926068947E-17,
-1.));
#16507=DIRECTION('ref_axis',(0.852431871234061,0.522838316216779,-3.69481373062586E-23));
#16508=DIRECTION('center_axis',(2.73022310513781E-17,-4.45132926068947E-17,
1.));
#16509=DIRECTION('ref_axis',(-0.852431871234064,-0.522838316216775,3.69481375527776E-23));
#16510=DIRECTION('center_axis',(-2.73022310513781E-17,4.45132926068947E-17,
-1.));
#16511=DIRECTION('ref_axis',(0.852431871234064,0.522838316216775,-3.69481375527776E-23));
#16512=DIRECTION('',(2.73022310513781E-17,-4.45132926068947E-17,1.));
#16513=DIRECTION('center_axis',(-2.73022310513781E-17,4.45132926068947E-17,
-1.));
#16514=DIRECTION('ref_axis',(0.852431871234064,0.522838316216775,-3.69481375527776E-23));
#16515=DIRECTION('center_axis',(2.73022310513781E-17,-4.45132926068947E-17,
1.));
#16516=DIRECTION('ref_axis',(-0.852431871234061,-0.522838316216779,3.69481373062586E-23));
#16517=DIRECTION('center_axis',(-2.73022310513781E-17,4.45132926068947E-17,
-1.));
#16518=DIRECTION('ref_axis',(0.852431871234061,0.522838316216779,-3.69481373062586E-23));
#16519=DIRECTION('',(2.73022310513781E-17,-4.45132926068947E-17,1.));
#16520=DIRECTION('center_axis',(-2.73022310513781E-17,4.45132926068947E-17,
-1.));
#16521=DIRECTION('ref_axis',(0.852431871234061,0.522838316216779,-3.69481373062586E-23));
#16522=DIRECTION('center_axis',(-0.852431871234063,-0.522838316216777,-2.44136686633116E-17));
#16523=DIRECTION('ref_axis',(-0.522838316216777,0.852431871234063,2.31111593326468E-32));
#16524=DIRECTION('center_axis',(0.852431871234063,0.522838316216777,2.44136686633116E-17));
#16525=DIRECTION('ref_axis',(0.522838316216777,-0.852431871234063,-2.31111593326468E-32));
#16526=DIRECTION('',(-0.852431871234063,-0.522838316216777,-2.44136686633116E-17));
#16527=DIRECTION('center_axis',(-0.852431871234063,-0.522838316216777,-2.44136686633116E-17));
#16528=DIRECTION('ref_axis',(-0.522838316216777,0.852431871234063,2.31111593326468E-32));
#16529=DIRECTION('',(0.852431871234063,0.522838316216777,2.44136686633116E-17));
#16530=DIRECTION('center_axis',(0.852431871234063,0.522838316216777,2.44136686633116E-17));
#16531=DIRECTION('ref_axis',(0.522838316216777,-0.852431871234063,3.23556230657056E-32));
#16532=DIRECTION('',(0.852431871234063,0.522838316216777,2.44136686633116E-17));
#16533=DIRECTION('center_axis',(0.852431871234063,0.522838316216777,2.44136686633116E-17));
#16534=DIRECTION('ref_axis',(0.522838316216777,-0.852431871234063,-2.31111593326468E-32));
#16535=DIRECTION('',(0.852431871234063,0.522838316216777,2.44136686633116E-17));
#16536=DIRECTION('center_axis',(0.852431871234063,0.522838316216777,2.44136686633116E-17));
#16537=DIRECTION('ref_axis',(0.522838316216777,-0.852431871234063,3.23556230657056E-32));
#16538=DIRECTION('',(-0.852431871234063,-0.522838316216777,-2.44136686633116E-17));
#16539=DIRECTION('center_axis',(-0.852431871234063,-0.522838316216777,-2.44136686633116E-17));
#16540=DIRECTION('ref_axis',(-0.522838316216777,0.852431871234063,2.31111593326468E-32));
#16541=DIRECTION('center_axis',(-0.852431871234063,-0.522838316216777,-2.44136686633116E-17));
#16542=DIRECTION('ref_axis',(-0.522838316216777,0.852431871234063,1.54074395550979E-32));
#16543=DIRECTION('center_axis',(0.852431871234063,0.522838316216777,2.44136686633116E-17));
#16544=DIRECTION('ref_axis',(0.522838316216777,-0.852431871234063,-1.54074395550979E-32));
#16545=DIRECTION('',(0.852431871234063,0.522838316216777,2.44136686633116E-17));
#16546=DIRECTION('center_axis',(-0.852431871234063,-0.522838316216777,-2.44136686633116E-17));
#16547=DIRECTION('ref_axis',(0.522838316216777,-0.852431871234063,-1.54074395550979E-32));
#16548=DIRECTION('',(0.852431871234063,0.522838316216777,2.44136686633116E-17));
#16549=DIRECTION('center_axis',(0.852431871234063,0.522838316216777,2.44136686633116E-17));
#16550=DIRECTION('ref_axis',(0.522838316216777,-0.852431871234063,-1.54074395550979E-32));
#16551=DIRECTION('center_axis',(-0.852431871234063,-0.522838316216777,-2.44136686633116E-17));
#16552=DIRECTION('ref_axis',(-0.522838316216777,0.852431871234063,1.54074395550979E-32));
#16553=DIRECTION('',(0.852431871234063,0.522838316216777,2.44136686633116E-17));
#16554=DIRECTION('center_axis',(0.852431871234063,0.522838316216777,2.44136686633116E-17));
#16555=DIRECTION('ref_axis',(0.522838316216777,-0.852431871234063,-1.54074395550979E-32));
#16556=DIRECTION('center_axis',(-0.852431871234063,-0.522838316216777,-2.44136686633116E-17));
#16557=DIRECTION('ref_axis',(-0.522838316216777,0.852431871234063,1.54074395550979E-32));
#16558=DIRECTION('center_axis',(-0.852431871234063,-0.522838316216777,-2.44136686633116E-17));
#16559=DIRECTION('ref_axis',(-0.522838316216777,0.852431871234063,1.54074395550979E-32));
#16560=DIRECTION('',(-0.852431871234063,-0.522838316216777,-2.44136686633116E-17));
#16561=DIRECTION('center_axis',(-0.852431871234063,-0.522838316216777,-2.44136686633116E-17));
#16562=DIRECTION('ref_axis',(0.522838316216777,-0.852431871234063,-1.54074395550979E-32));
#16563=DIRECTION('',(0.852431871234063,0.522838316216777,2.44136686633116E-17));
#16564=DIRECTION('center_axis',(-0.522838316216777,0.852431871234063,1.10549867763274E-16));
#16565=DIRECTION('ref_axis',(0.852431871234063,0.522838316216777,2.44136686633116E-17));
#16566=DIRECTION('',(-0.852431871234063,-0.522838316216777,-2.44136686633116E-17));
#16567=DIRECTION('',(2.73022310513781E-17,-4.45132926068947E-17,1.));
#16568=DIRECTION('',(-0.852431871234063,-0.522838316216777,-2.44136686633116E-17));
#16569=DIRECTION('',(2.73022310513781E-17,-4.45132926068947E-17,1.));
#16570=DIRECTION('center_axis',(0.522838316216777,-0.852431871234063,-1.10549867763274E-16));
#16571=DIRECTION('ref_axis',(-0.852431871234063,-0.522838316216777,-2.44136686633116E-17));
#16572=DIRECTION('',(2.73022310513781E-17,-4.45132926068947E-17,1.));
#16573=DIRECTION('',(-0.852431871234063,-0.522838316216777,-2.44136686633116E-17));
#16574=DIRECTION('',(-2.73022310513781E-17,4.45132926068947E-17,-1.));
#16575=DIRECTION('',(-0.852431871234063,-0.522838316216777,-2.44136686633116E-17));
#16576=DIRECTION('center_axis',(-0.852431871234063,-0.522838316216777,-2.44136686633116E-17));
#16577=DIRECTION('ref_axis',(-0.522838316216777,0.852431871234063,1.10549867763274E-16));
#16578=DIRECTION('',(0.522838316216777,-0.852431871234063,-1.10549867763274E-16));
#16579=DIRECTION('',(0.522838316216777,-0.852431871234063,-1.10549867763274E-16));
#16580=DIRECTION('center_axis',(0.852431871234063,0.522838316216777,2.44136686633116E-17));
#16581=DIRECTION('ref_axis',(0.522838316216777,-0.852431871234063,-1.10549867763274E-16));
#16582=DIRECTION('center_axis',(-0.852431871234063,-0.522838316216777,-2.44136686633116E-17));
#16583=DIRECTION('ref_axis',(-0.522838316216777,0.852431871234063,1.10549867763274E-16));
#16584=DIRECTION('',(0.522838316216777,-0.852431871234063,-1.10549867763274E-16));
#16585=DIRECTION('',(0.522838316216777,-0.852431871234063,-1.10549867763274E-16));
#16586=DIRECTION('',(2.73022310513781E-17,-4.45132926068947E-17,1.));
#16587=DIRECTION('center_axis',(-0.522838316216777,0.852431871234063,1.10549867763274E-16));
#16588=DIRECTION('ref_axis',(0.852431871234063,0.522838316216777,2.44136686633116E-17));
#16589=DIRECTION('',(-0.852431871234063,-0.522838316216777,-2.44136686633116E-17));
#16590=DIRECTION('',(2.73022310513781E-17,-4.45132926068947E-17,1.));
#16591=DIRECTION('',(-0.852431871234063,-0.522838316216777,-2.44136686633116E-17));
#16592=DIRECTION('center_axis',(-0.253157481559667,0.967425082128,1.12879065814692E-16));
#16593=DIRECTION('ref_axis',(0.967425082128,0.253157481559667,-8.69580248635087E-18));
#16594=DIRECTION('',(-0.967425082128,-0.253157481559667,8.69580248635087E-18));
#16595=DIRECTION('',(2.73022310513781E-17,-4.45132926068947E-17,1.));
#16596=DIRECTION('',(-0.967425082128,-0.253157481559667,8.69580248635087E-18));
#16597=DIRECTION('center_axis',(-0.852431871234063,-0.522838316216777,-2.44136686633116E-17));
#16598=DIRECTION('ref_axis',(-0.522838316216777,0.852431871234063,1.10549867763274E-16));
#16599=DIRECTION('',(0.522838316216777,-0.852431871234063,-1.10549867763274E-16));
#16600=DIRECTION('',(0.522838316216777,-0.852431871234063,-1.10549867763274E-16));
#16601=DIRECTION('center_axis',(-6.49121029325306E-18,5.72777133413967E-17,
-1.));
#16602=DIRECTION('ref_axis',(0.852431871234063,0.522838316216777,2.44136686633116E-17));
#16603=DIRECTION('center_axis',(-6.49121029325306E-18,5.72777133413967E-17,
-1.));
#16604=DIRECTION('ref_axis',(0.852431871234063,0.522838316216777,2.44136686633116E-17));
#16605=DIRECTION('center_axis',(0.852431871234063,0.522838316216777,2.44136686633116E-17));
#16606=DIRECTION('ref_axis',(0.522838316216777,-0.852431871234063,-1.10549867763274E-16));
#16607=DIRECTION('',(0.522838316216777,-0.852431871234063,-1.10549867763274E-16));
#16608=DIRECTION('',(-2.73022310513781E-17,4.45132926068947E-17,-1.));
#16609=DIRECTION('',(0.522838316216777,-0.852431871234063,-1.10549867763274E-16));
#16610=DIRECTION('center_axis',(0.522838316216777,-0.852431871234063,-1.10549867763274E-16));
#16611=DIRECTION('ref_axis',(-0.852431871234063,-0.522838316216777,-2.44136686633116E-17));
#16612=DIRECTION('',(-0.852431871234063,-0.522838316216777,-2.44136686633116E-17));
#16613=DIRECTION('',(-0.852431871234063,-0.522838316216777,-2.44136686633116E-17));
#16614=DIRECTION('',(-2.73022310513781E-17,4.45132926068947E-17,-1.));
#16615=DIRECTION('center_axis',(0.852431871234063,0.522838316216777,2.44136686633116E-17));
#16616=DIRECTION('ref_axis',(0.522838316216777,-0.852431871234063,-1.10549867763274E-16));
#16617=DIRECTION('',(0.522838316216777,-0.852431871234063,-1.10549867763274E-16));
#16618=DIRECTION('',(-2.73022310513781E-17,4.45132926068947E-17,-1.));
#16619=DIRECTION('',(0.522838316216777,-0.852431871234063,-1.10549867763274E-16));
#16620=DIRECTION('center_axis',(0.253157481559667,-0.967425082128,-1.12879065814692E-16));
#16621=DIRECTION('ref_axis',(-0.967425082128,-0.253157481559667,8.69580248635087E-18));
#16622=DIRECTION('',(-0.967425082128,-0.253157481559667,8.69580248635087E-18));
#16623=DIRECTION('',(-0.967425082128,-0.253157481559667,8.69580248635087E-18));
#16624=DIRECTION('center_axis',(6.49121029325306E-18,-5.72777133413967E-17,
1.));
#16625=DIRECTION('ref_axis',(0.852431871234063,0.522838316216777,2.44136686633116E-17));
#16626=DIRECTION('center_axis',(6.49121029325306E-18,-5.72777133413967E-17,
1.));
#16627=DIRECTION('ref_axis',(0.852431871234063,0.522838316216777,2.44136686633116E-17));
#16628=DIRECTION('center_axis',(0.852431871234063,0.522838316216777,2.44136686633116E-17));
#16629=DIRECTION('ref_axis',(-0.522838316216777,0.852431871234063,3.21624529935327E-16));
#16630=DIRECTION('center_axis',(0.852431871234063,0.522838316216777,2.44136686633116E-17));
#16631=DIRECTION('ref_axis',(0.522838316216777,-0.852431871234063,1.69481835106077E-32));
#16632=DIRECTION('center_axis',(0.852431871234063,0.522838316216777,2.44136686633116E-17));
#16633=DIRECTION('ref_axis',(0.522838316216777,-0.852431871234063,-6.16297582203915E-33));
#16634=DIRECTION('center_axis',(0.852431871234063,0.522838316216777,2.44136686633116E-17));
#16635=DIRECTION('ref_axis',(-0.522838316216777,0.852431871234063,1.89882151931499E-15));
#16636=DIRECTION('center_axis',(-0.852431871234063,-0.522838316216777,-2.44136686633116E-17));
#16637=DIRECTION('ref_axis',(0.522838316216777,-0.852431871234063,3.08148791101958E-33));
#16638=DIRECTION('center_axis',(0.852431871234063,0.522838316216777,2.44136686633116E-17));
#16639=DIRECTION('ref_axis',(0.522838316216777,-0.852431871234063,-1.10549867763274E-16));
#16640=DIRECTION('center_axis',(0.852431871234063,0.522838316216777,2.44136686633116E-17));
#16641=DIRECTION('ref_axis',(0.522838316216777,-0.852431871234063,-1.10549867763274E-16));
#16642=DIRECTION('center_axis',(0.852431871234063,0.522838316216777,2.44136686633116E-17));
#16643=DIRECTION('ref_axis',(-0.522838316216777,0.852431871234062,-3.45797464736582E-13));
#22547=CARTESIAN_POINT('',(0.,0.,0.));
#22548=CARTESIAN_POINT('Origin',(239.288983046696,153.123984191663,272.073593133703));
#22549=CARTESIAN_POINT('',(235.453039626143,150.771211768687,272.073593133703));
#22550=CARTESIAN_POINT('Origin',(239.288983046696,153.123984191663,272.073593133703));
#22551=CARTESIAN_POINT('',(235.453039626143,150.771211768687,270.073593133703));
#22552=CARTESIAN_POINT('',(235.453039626143,150.771211768687,272.073593133703));
#22553=CARTESIAN_POINT('Origin',(239.288983046696,153.123984191663,270.073593133703));
#22554=CARTESIAN_POINT('Origin',(272.715792356497,163.654816037544,272.073593133703));
#22555=CARTESIAN_POINT('',(268.453633000327,161.04062445646,272.073593133703));
#22556=CARTESIAN_POINT('Origin',(272.715792356497,163.654816037544,272.073593133703));
#22557=CARTESIAN_POINT('',(268.453633000327,161.04062445646,270.073593133703));
#22558=CARTESIAN_POINT('',(268.453633000327,161.04062445646,272.073593133703));
#22559=CARTESIAN_POINT('Origin',(272.715792356497,163.654816037544,270.073593133703));
#22560=CARTESIAN_POINT('Origin',(239.288983046696,153.123984191663,248.073593133703));
#22561=CARTESIAN_POINT('',(243.12492646725,155.476756614638,248.073593133703));
#22562=CARTESIAN_POINT('Origin',(239.288983046696,153.123984191663,248.073593133703));
#22563=CARTESIAN_POINT('',(243.12492646725,155.476756614638,250.073593133703));
#22564=CARTESIAN_POINT('',(243.12492646725,155.476756614638,248.073593133703));
#22565=CARTESIAN_POINT('Origin',(239.288983046696,153.123984191663,250.073593133703));
#22566=CARTESIAN_POINT('Origin',(272.715792356497,163.654816037544,248.073593133703));
#22567=CARTESIAN_POINT('',(276.977951712667,166.269007618627,248.073593133703));
#22568=CARTESIAN_POINT('Origin',(272.715792356497,163.654816037544,248.073593133703));
#22569=CARTESIAN_POINT('',(276.977951712667,166.269007618627,250.073593133703));
#22570=CARTESIAN_POINT('',(276.977951712667,166.269007618627,248.073593133703));
#22571=CARTESIAN_POINT('Origin',(272.715792356497,163.654816037544,250.073593133703));
#22572=CARTESIAN_POINT('Origin',(297.208732752758,202.139824427113,260.073593133703));
#22573=CARTESIAN_POINT('',(302.437115914926,193.615505714772,260.073593133703));
#22574=CARTESIAN_POINT('Origin',(297.208732752758,202.139824427113,260.073593133703));
#22575=CARTESIAN_POINT('',(280.27388726284,180.021709493136,260.073593133703));
#22576=CARTESIAN_POINT('',(302.437115914926,193.615505714772,260.073593133703));
#22577=CARTESIAN_POINT('',(275.045504100673,188.546028205476,270.073593133703));
#22578=CARTESIAN_POINT('Origin',(275.045504100673,188.546028205476,260.073593133703));
#22579=CARTESIAN_POINT('',(239.243365508842,166.586818924372,270.073593133703));
#22580=CARTESIAN_POINT('',(297.208732752758,202.139824427113,270.073593133703));
#22581=CARTESIAN_POINT('',(236.629173927758,170.848978280542,268.733847171548));
#22582=CARTESIAN_POINT('Origin',(239.243365508842,166.586818924372,260.073593133703));
#22583=CARTESIAN_POINT('',(253.677811352439,181.305744604878,268.733847171548));
#22584=CARTESIAN_POINT('',(236.629173927758,170.848978280542,268.733847171548));
#22585=CARTESIAN_POINT('',(253.677811352439,181.305744604878,251.413339095859));
#22586=CARTESIAN_POINT('Origin',(256.292002933523,177.043585248707,260.073593133703));
#22587=CARTESIAN_POINT('',(236.629173927758,170.848978280542,251.413339095859));
#22588=CARTESIAN_POINT('',(236.629173927758,170.848978280542,251.413339095859));
#22589=CARTESIAN_POINT('',(239.243365508842,166.586818924372,250.073593133703));
#22590=CARTESIAN_POINT('Origin',(239.243365508842,166.586818924372,260.073593133703));
#22591=CARTESIAN_POINT('',(275.045504100673,188.546028205476,250.073593133703));
#22592=CARTESIAN_POINT('',(297.208732752758,202.139824427113,250.073593133703));
#22593=CARTESIAN_POINT('Origin',(275.045504100673,188.546028205476,260.073593133703));
#22594=CARTESIAN_POINT('Origin',(297.208732752758,202.139824427113,260.073593133703));
#22595=CARTESIAN_POINT('',(255.323361884785,182.448125072191,249.2175955373));
#22596=CARTESIAN_POINT('',(255.323361884814,182.448125072217,270.929590730103));
#22597=CARTESIAN_POINT('Origin',(257.996866675991,178.089261881141,260.073593133703));
#22598=CARTESIAN_POINT('',(255.058804871611,182.152775729166,270.982305248339));
#22599=CARTESIAN_POINT('Ctrl Pts',(255.323361885007,182.448125072171,270.929590730169));
#22600=CARTESIAN_POINT('Ctrl Pts',(255.309569700968,182.408536079969,270.942089768565));
#22601=CARTESIAN_POINT('Ctrl Pts',(255.289379287412,182.371026850316,270.952064384874));
#22602=CARTESIAN_POINT('Ctrl Pts',(255.26450099475,182.336243715935,270.959783119772));
#22603=CARTESIAN_POINT('Ctrl Pts',(255.250346319745,182.316453613395,270.964174746858));
#22604=CARTESIAN_POINT('Ctrl Pts',(255.234674366869,182.297545581916,270.967835176688));
#22605=CARTESIAN_POINT('Ctrl Pts',(255.217801828123,182.279635918025,270.970807219426));
#22606=CARTESIAN_POINT('Ctrl Pts',(255.183565204112,182.243294829227,270.976837889219));
#22607=CARTESIAN_POINT('Ctrl Pts',(255.145217910695,182.21112323878,270.980215787129));
#22608=CARTESIAN_POINT('Ctrl Pts',(255.104099246087,182.182404890805,270.981583115665));
#22609=CARTESIAN_POINT('Ctrl Pts',(255.089337425425,182.17209485018,270.982073993928));
#22610=CARTESIAN_POINT('Ctrl Pts',(255.07421853595,182.16222968627,270.982305248323));
#22611=CARTESIAN_POINT('Ctrl Pts',(255.058804871611,182.152775729166,270.982305248339));
#22612=CARTESIAN_POINT('',(236.629173927758,170.848978280542,270.982305248339));
#22613=CARTESIAN_POINT('',(236.629173927758,170.848978280542,270.982305248339));
#22614=CARTESIAN_POINT('',(239.243365508842,166.586818924372,272.073593133703));
#22615=CARTESIAN_POINT('Origin',(239.243365508842,166.586818924372,260.073593133703));
#22616=CARTESIAN_POINT('',(275.045504100673,188.546028205476,272.073593133703));
#22617=CARTESIAN_POINT('',(297.208732752758,202.139824427113,272.073593133703));
#22618=CARTESIAN_POINT('',(278.513621142497,182.891634853029,270.073593133703));
#22619=CARTESIAN_POINT('Origin',(275.045504100673,188.546028205476,260.073593133703));
#22620=CARTESIAN_POINT('',(281.319563895274,178.316845750668,260.073593133703));
#22621=CARTESIAN_POINT('Origin',(275.045504100673,188.546028205476,260.073593133703));
#22622=CARTESIAN_POINT('',(303.48279254736,191.910641972304,260.073593133703));
#22623=CARTESIAN_POINT('',(303.48279254736,191.910641972304,260.073593133703));
#22624=CARTESIAN_POINT('Origin',(297.208732752758,202.139824427113,260.073593133703));
#22625=CARTESIAN_POINT('',(278.513621142497,182.891634853029,250.073593133703));
#22626=CARTESIAN_POINT('Origin',(275.045504100673,188.546028205476,260.073593133703));
#22627=CARTESIAN_POINT('',(275.045504100673,188.546028205476,248.073593133703));
#22628=CARTESIAN_POINT('Origin',(275.045504100673,188.546028205476,260.073593133703));
#22629=CARTESIAN_POINT('',(239.243365508842,166.586818924372,248.073593133703));
#22630=CARTESIAN_POINT('',(297.208732752758,202.139824427113,248.073593133703));
#22631=CARTESIAN_POINT('',(236.629173927758,170.848978280542,249.164881019068));
#22632=CARTESIAN_POINT('Origin',(239.243365508842,166.586818924372,260.073593133703));
#22633=CARTESIAN_POINT('',(255.058804871617,182.152775729169,249.164881019068));
#22634=CARTESIAN_POINT('',(236.629173927758,170.848978280542,249.164881019068));
#22635=CARTESIAN_POINT('Ctrl Pts',(255.058804871617,182.152775729169,249.164881019068));
#22636=CARTESIAN_POINT('Ctrl Pts',(255.102027325485,182.179286182221,249.164881019113));
#22637=CARTESIAN_POINT('Ctrl Pts',(255.142563428073,182.208749139151,249.166674552376));
#22638=CARTESIAN_POINT('Ctrl Pts',(255.179508383441,182.24215669622,249.170886992558));
#22639=CARTESIAN_POINT('Ctrl Pts',(255.1926006349,182.253995393369,249.172379762696));
#22640=CARTESIAN_POINT('Ctrl Pts',(255.205242003714,182.26632930192,249.174176678126));
#22641=CARTESIAN_POINT('Ctrl Pts',(255.217392602471,182.279201956245,249.176307129975));
#22642=CARTESIAN_POINT('Ctrl Pts',(255.249844358091,182.313582174103,249.181997129631));
#22643=CARTESIAN_POINT('Ctrl Pts',(255.278272607663,182.352497583317,249.190460078823));
#22644=CARTESIAN_POINT('Ctrl Pts',(255.299732473223,182.393719901414,249.201635214537));
#22645=CARTESIAN_POINT('Ctrl Pts',(255.308981574346,182.411486526629,249.20645164547));
#22646=CARTESIAN_POINT('Ctrl Pts',(255.316936407192,182.429681419483,249.211772506003));
#22647=CARTESIAN_POINT('Ctrl Pts',(255.323361884996,182.448125072141,249.217595537228));
#22648=CARTESIAN_POINT('Origin',(256.292002933523,177.043585248707,248.073593133703));
#22649=CARTESIAN_POINT('',(225.604455569097,158.221405864903,250.073593133703));
#22650=CARTESIAN_POINT('',(256.292002933523,177.043585248707,250.073593133703));
#22651=CARTESIAN_POINT('',(239.243365508842,166.586818924372,248.073593133703));
#22652=CARTESIAN_POINT('',(225.604455569097,158.221405864903,248.073593133703));
#22653=CARTESIAN_POINT('',(256.292002933523,177.043585248707,248.073593133703));
#22654=CARTESIAN_POINT('',(225.604455569097,158.221405864903,248.073593133703));
#22655=CARTESIAN_POINT('Origin',(256.292002933523,177.043585248707,272.073593133703));
#22656=CARTESIAN_POINT('',(239.243365508842,166.586818924372,270.073593133703));
#22657=CARTESIAN_POINT('',(225.604455569097,158.221405864903,270.073593133703));
#22658=CARTESIAN_POINT('',(256.292002933523,177.043585248707,270.073593133703));
#22659=CARTESIAN_POINT('',(225.604455569097,158.221405864903,272.073593133703));
#22660=CARTESIAN_POINT('',(225.604455569097,158.221405864903,272.073593133703));
#22661=CARTESIAN_POINT('',(256.292002933523,177.043585248707,272.073593133703));
#22662=CARTESIAN_POINT('Origin',(275.045504100673,188.546028205476,230.073593133703));
#22663=CARTESIAN_POINT('',(275.045504100673,188.546028205476,270.073593133703));
#22664=CARTESIAN_POINT('',(275.045504100673,188.546028205476,250.073593133703));
#22665=CARTESIAN_POINT('Origin',(297.208732752758,202.139824427113,260.073593133703));
#22666=CARTESIAN_POINT('Origin',(275.045504100673,188.546028205476,248.073593133703));
#22667=CARTESIAN_POINT('',(289.684976954742,164.677935810923,248.073593133703));
#22668=CARTESIAN_POINT('',(275.045504100673,188.546028205476,248.073593133703));
#22669=CARTESIAN_POINT('',(289.684976954742,164.677935810923,250.073593133703));
#22670=CARTESIAN_POINT('',(275.045504100673,188.546028205476,250.073593133703));
#22671=CARTESIAN_POINT('',(289.684976954742,164.677935810923,248.073593133703));
#22672=CARTESIAN_POINT('Origin',(270.931475787593,153.175492854154,248.073593133703));
#22673=CARTESIAN_POINT('',(268.374180173891,151.606977905503,250.073593133703));
#22674=CARTESIAN_POINT('',(270.931475787593,153.175492854154,250.073593133703));
#22675=CARTESIAN_POINT('',(268.374180173891,151.606977905503,248.073593133703));
#22676=CARTESIAN_POINT('',(268.374180173891,151.606977905503,248.073593133703));
#22677=CARTESIAN_POINT('',(270.931475787593,153.175492854154,248.073593133703));
#22678=CARTESIAN_POINT('Origin',(263.296036423484,150.278120398498,248.073593133703));
#22679=CARTESIAN_POINT('',(235.015545260999,142.87763218269,250.073593133703));
#22680=CARTESIAN_POINT('',(263.296036423484,150.278120398498,250.073593133703));
#22681=CARTESIAN_POINT('',(235.015545260999,142.87763218269,248.073593133703));
#22682=CARTESIAN_POINT('',(235.015545260999,142.87763218269,248.073593133703));
#22683=CARTESIAN_POINT('',(263.296036423484,150.278120398498,248.073593133703));
#22684=CARTESIAN_POINT('Origin',(225.604455569097,158.221405864903,248.073593133703));
#22685=CARTESIAN_POINT('',(225.604455569097,158.221405864903,250.073593133703));
#22686=CARTESIAN_POINT('',(225.604455569097,158.221405864903,248.073593133703));
#22687=CARTESIAN_POINT('Origin',(256.292002933523,177.043585248707,248.073593133703));
#22688=CARTESIAN_POINT('Origin',(256.292002933523,177.043585248707,250.073593133703));
#22689=CARTESIAN_POINT('Origin',(275.045504100673,188.546028205476,272.073593133703));
#22690=CARTESIAN_POINT('',(289.684976954742,164.677935810923,272.073593133703));
#22691=CARTESIAN_POINT('',(275.045504100673,188.546028205476,272.073593133703));
#22692=CARTESIAN_POINT('',(289.684976954742,164.677935810923,270.073593133703));
#22693=CARTESIAN_POINT('',(289.684976954742,164.677935810923,272.073593133703));
#22694=CARTESIAN_POINT('',(275.045504100673,188.546028205476,270.073593133703));
#22695=CARTESIAN_POINT('Origin',(270.931475787593,153.175492854154,272.073593133703));
#22696=CARTESIAN_POINT('',(268.374180173891,151.606977905503,270.073593133703));
#22697=CARTESIAN_POINT('',(270.931475787593,153.175492854154,270.073593133703));
#22698=CARTESIAN_POINT('',(268.374180173891,151.606977905503,272.073593133703));
#22699=CARTESIAN_POINT('',(270.931475787593,153.175492854154,272.073593133703));
#22700=CARTESIAN_POINT('',(268.374180173891,151.606977905503,272.073593133703));
#22701=CARTESIAN_POINT('Origin',(225.604455569097,158.221405864903,272.073593133703));
#22702=CARTESIAN_POINT('',(235.015545260999,142.87763218269,270.073593133703));
#22703=CARTESIAN_POINT('',(225.604455569097,158.221405864903,270.073593133703));
#22704=CARTESIAN_POINT('',(235.015545260999,142.87763218269,272.073593133703));
#22705=CARTESIAN_POINT('',(235.015545260999,142.87763218269,272.073593133703));
#22706=CARTESIAN_POINT('',(225.604455569097,158.221405864903,272.073593133703));
#22707=CARTESIAN_POINT('Origin',(263.296036423484,150.278120398498,272.073593133703));
#22708=CARTESIAN_POINT('',(263.296036423484,150.278120398498,270.073593133703));
#22709=CARTESIAN_POINT('',(263.296036423484,150.278120398498,272.073593133703));
#22710=CARTESIAN_POINT('Origin',(256.292002933523,177.043585248707,272.073593133703));
#22711=CARTESIAN_POINT('Origin',(256.292002933523,177.043585248707,270.073593133703));
#22712=CARTESIAN_POINT('Origin',(249.999939717625,149.049376857752,260.073593133703));
#22713=CARTESIAN_POINT('Origin',(267.048577142306,159.506143182087,260.073593133703));
#22714=CARTESIAN_POINT('Origin',(249.999939717625,149.049376857752,260.073593133703));
#22715=CARTESIAN_POINT('Origin',(240.326199116368,164.821374714051,260.073593133703));
#22716=CARTESIAN_POINT('Ctrl Pts',(255.058804869969,182.152775728158,270.982305248339));
#22717=CARTESIAN_POINT('Ctrl Pts',(254.922595243703,182.147186996158,270.939231074838));
#22718=CARTESIAN_POINT('Ctrl Pts',(254.792319846723,182.1678785851,270.882674845301));
#22719=CARTESIAN_POINT('Ctrl Pts',(254.547149308436,182.228970127669,270.760014729386));
#22720=CARTESIAN_POINT('Ctrl Pts',(254.430102458011,182.270513662175,270.692574498549));
#22721=CARTESIAN_POINT('Ctrl Pts',(254.091846405705,182.411381584387,270.478647373104));
#22722=CARTESIAN_POINT('Ctrl Pts',(253.888226908793,182.52392263632,270.324232289594));
#22723=CARTESIAN_POINT('Ctrl Pts',(253.503176846748,182.759323529108,269.997439492304));
#22724=CARTESIAN_POINT('Ctrl Pts',(253.322509839,182.883112909143,269.824845969452));
#22725=CARTESIAN_POINT('Ctrl Pts',(252.978070665713,183.133913082514,269.462735650107));
#22726=CARTESIAN_POINT('Ctrl Pts',(252.814019303634,183.261450177997,269.272569866411));
#22727=CARTESIAN_POINT('Ctrl Pts',(252.349393784202,183.637467244233,268.685694556367));
#22728=CARTESIAN_POINT('Ctrl Pts',(252.073664492895,183.880694398784,268.270651629051));
#22729=CARTESIAN_POINT('Ctrl Pts',(251.574095308201,184.338327118907,267.395153694069));
#22730=CARTESIAN_POINT('Ctrl Pts',(251.350598392334,184.553055890188,266.934666983117));
#22731=CARTESIAN_POINT('Ctrl Pts',(251.050673609181,184.84821394174,266.209201808336));
#22732=CARTESIAN_POINT('Ctrl Pts',(250.956756662856,184.942020874301,265.961675454384));
#22733=CARTESIAN_POINT('Ctrl Pts',(250.782916004701,185.117468763908,265.462143203401));
#22734=CARTESIAN_POINT('Ctrl Pts',(250.702618023797,185.199479981665,265.20926576918));
#22735=CARTESIAN_POINT('Ctrl Pts',(250.480600808949,185.428075012049,264.44146848943));
#22736=CARTESIAN_POINT('Ctrl Pts',(250.357646619975,185.557264701136,263.917422833903));
#22737=CARTESIAN_POINT('Ctrl Pts',(250.159716763548,185.766878090088,262.844897070672));
#22738=CARTESIAN_POINT('Ctrl Pts',(250.084593037062,185.847495973639,262.293315498942));
#22739=CARTESIAN_POINT('Ctrl Pts',(249.98515941521,185.95447401283,261.184983142805));
#22740=CARTESIAN_POINT('Ctrl Pts',(249.960387400451,185.981329584333,260.62741827262));
#22741=CARTESIAN_POINT('Ctrl Pts',(249.96100832076,185.98065816754,258.945148252925));
#22742=CARTESIAN_POINT('Ctrl Pts',(250.059575673001,185.872958537603,257.848516427325));
#22743=CARTESIAN_POINT('Ctrl Pts',(250.355456958999,185.559569730516,256.239858184419));
#22744=CARTESIAN_POINT('Ctrl Pts',(250.480425610475,185.42824964895,255.706112477511));
#22745=CARTESIAN_POINT('Ctrl Pts',(250.777739784718,185.122138321099,254.678340409923));
#22746=CARTESIAN_POINT('Ctrl Pts',(250.949992239702,184.947355826575,254.182401072184));
#22747=CARTESIAN_POINT('Ctrl Pts',(251.344711962776,184.558789117574,253.225886058467));
#22748=CARTESIAN_POINT('Ctrl Pts',(251.567066041168,184.344908180937,252.765302871011));
#22749=CARTESIAN_POINT('Ctrl Pts',(252.070625488688,183.883339233532,251.880927869941));
#22750=CARTESIAN_POINT('Ctrl Pts',(252.350194703928,183.63679940324,251.460417476297));
#22751=CARTESIAN_POINT('Ctrl Pts',(252.814261793661,183.261263785637,250.874341464003));
#22752=CARTESIAN_POINT('Ctrl Pts',(252.976797851985,183.134875023001,250.685864335876));
#22753=CARTESIAN_POINT('Ctrl Pts',(253.321579334035,182.883755518574,250.323243418964));
#22754=CARTESIAN_POINT('Ctrl Pts',(253.503980821481,182.758747305024,250.148944925558));
#22755=CARTESIAN_POINT('Ctrl Pts',(253.890944404526,182.522346778811,249.820768240594));
#22756=CARTESIAN_POINT('Ctrl Pts',(254.096402914617,182.409199663039,249.665403438688));
#22757=CARTESIAN_POINT('Ctrl Pts',(254.432638579187,182.26960273328,249.45313743041));
#22758=CARTESIAN_POINT('Ctrl Pts',(254.548686887323,182.228477031682,249.386324330007));
#22759=CARTESIAN_POINT('Ctrl Pts',(254.793947631671,182.167584364359,249.263775994265));
#22760=CARTESIAN_POINT('Ctrl Pts',(254.9238364217,182.147237922157,249.207562689353));
#22761=CARTESIAN_POINT('Ctrl Pts',(255.058804869969,182.152775728158,249.164881019068));
#22762=CARTESIAN_POINT('Origin',(240.326199116368,164.821374714051,260.073593133703));
#22763=CARTESIAN_POINT('Origin',(239.243365508842,166.586818924372,260.073593133703));
#22764=CARTESIAN_POINT('Origin',(256.292002933523,177.043585248707,260.073593133703));
#22765=CARTESIAN_POINT('Origin',(257.996866675991,178.089261881141,260.073593133703));
#22766=CARTESIAN_POINT('Ctrl Pts',(255.32336188472,182.448125072297,249.217595537359));
#22767=CARTESIAN_POINT('Ctrl Pts',(255.305592473701,182.437226220217,249.217595537395));
#22768=CARTESIAN_POINT('Ctrl Pts',(255.286198795864,182.43009894237,249.219874591516));
#22769=CARTESIAN_POINT('Ctrl Pts',(255.266403935544,182.425927343183,249.223717258111));
#22770=CARTESIAN_POINT('Ctrl Pts',(255.251968219503,182.422885138271,249.22651958371));
#22771=CARTESIAN_POINT('Ctrl Pts',(255.237318898632,182.421415083184,249.230152526266));
#22772=CARTESIAN_POINT('Ctrl Pts',(255.222924497431,182.421205660522,249.23432258769));
#22773=CARTESIAN_POINT('Ctrl Pts',(255.203424097226,182.420921951205,249.239971858231));
#22774=CARTESIAN_POINT('Ctrl Pts',(255.184565977027,182.422652171011,249.246434572775));
#22775=CARTESIAN_POINT('Ctrl Pts',(255.166141185898,182.425740259873,249.253443856627));
#22776=CARTESIAN_POINT('Ctrl Pts',(255.152316064946,182.42805742058,249.258703302791));
#22777=CARTESIAN_POINT('Ctrl Pts',(255.138735222325,182.431138529906,249.264271900505));
#22778=CARTESIAN_POINT('Ctrl Pts',(255.125314763442,182.43469985398,249.270053972538));
#22779=CARTESIAN_POINT('Ctrl Pts',(255.098342238399,182.441857426132,249.281674818298));
#22780=CARTESIAN_POINT('Ctrl Pts',(255.072193027228,182.450958116289,249.294100019898));
#22781=CARTESIAN_POINT('Ctrl Pts',(255.046747612105,182.461389632585,249.307045409399));
#22782=CARTESIAN_POINT('Ctrl Pts',(255.018207282478,182.47308992956,249.321565340857));
#22783=CARTESIAN_POINT('Ctrl Pts',(254.99055223487,182.486464125929,249.336740338357));
#22784=CARTESIAN_POINT('Ctrl Pts',(254.963629642091,182.50062736719,249.352228706564));
#22785=CARTESIAN_POINT('Ctrl Pts',(254.958836407747,182.503148956956,249.354986218778));
#22786=CARTESIAN_POINT('Ctrl Pts',(254.954066429165,182.505695517326,249.357753784772));
#22787=CARTESIAN_POINT('Ctrl Pts',(254.949318892957,182.508262007514,249.360529620813));
#22788=CARTESIAN_POINT('Ctrl Pts',(254.913127437292,182.527826895861,249.381690396129));
#22789=CARTESIAN_POINT('Ctrl Pts',(254.878128477634,182.548688694715,249.403418625613));
#22790=CARTESIAN_POINT('Ctrl Pts',(254.844070018945,182.570521714466,249.425585370033));
#22791=CARTESIAN_POINT('Ctrl Pts',(254.80655594336,182.594569941682,249.450001182071));
#22792=CARTESIAN_POINT('Ctrl Pts',(254.770182649824,182.619796322315,249.474949455971));
#22793=CARTESIAN_POINT('Ctrl Pts',(254.734633012517,182.645744317309,249.500318724675));
#22794=CARTESIAN_POINT('Ctrl Pts',(254.704026539747,182.668084252745,249.522160405508));
#22795=CARTESIAN_POINT('Ctrl Pts',(254.67403095503,182.690958613402,249.544315530662));
#22796=CARTESIAN_POINT('Ctrl Pts',(254.644455404621,182.714066428366,249.566739565019));
#22797=CARTESIAN_POINT('Ctrl Pts',(254.590341043457,182.756346779108,249.607768802926));
#22798=CARTESIAN_POINT('Ctrl Pts',(254.537722157117,182.799604455555,249.649719683728));
#22799=CARTESIAN_POINT('Ctrl Pts',(254.486359613436,182.843564713015,249.692468853766));
#22800=CARTESIAN_POINT('Ctrl Pts',(254.432095924541,182.890008007361,249.737632654023));
#22801=CARTESIAN_POINT('Ctrl Pts',(254.379234258228,182.937235353287,249.783688222526));
#22802=CARTESIAN_POINT('Ctrl Pts',(254.327512963319,182.984905076776,249.830544503696));
#22803=CARTESIAN_POINT('Ctrl Pts',(254.271481709556,183.036547139845,249.881305339928));
#22804=CARTESIAN_POINT('Ctrl Pts',(254.216788466965,183.088708348173,249.933006591772));
#22805=CARTESIAN_POINT('Ctrl Pts',(254.163128675427,183.140935448316,249.985582995045));
#22806=CARTESIAN_POINT('Ctrl Pts',(254.148390615218,183.155280009194,250.000023494621));
#22807=CARTESIAN_POINT('Ctrl Pts',(254.133730683178,183.169629439894,250.014530251569));
#22808=CARTESIAN_POINT('Ctrl Pts',(254.119142948937,183.183974129141,250.02910240567));
#22809=CARTESIAN_POINT('Ctrl Pts',(254.037485369745,183.26427121838,250.110672772103));
#22810=CARTESIAN_POINT('Ctrl Pts',(253.958095813474,183.344700205996,250.194375829466));
#22811=CARTESIAN_POINT('Ctrl Pts',(253.880756017281,183.424975212899,250.280039742912));
#22812=CARTESIAN_POINT('Ctrl Pts',(253.798855156596,183.50998438645,250.370755630284));
#22813=CARTESIAN_POINT('Ctrl Pts',(253.719252476785,183.594820876681,250.463671450877));
#22814=CARTESIAN_POINT('Ctrl Pts',(253.641713921974,183.67913063593,250.558639388367));
#22815=CARTESIAN_POINT('Ctrl Pts',(253.556712663608,183.77155479377,250.662747521549));
#22816=CARTESIAN_POINT('Ctrl Pts',(253.474191353476,183.863346039261,250.769322888701));
#22817=CARTESIAN_POINT('Ctrl Pts',(253.393880298491,183.954020152393,250.878219862291));
#22818=CARTESIAN_POINT('Ctrl Pts',(253.340219189988,184.014605502991,250.950981106886));
#22819=CARTESIAN_POINT('Ctrl Pts',(253.287545690091,184.074691736403,251.024779800913));
#22820=CARTESIAN_POINT('Ctrl Pts',(253.2357893457,184.13413038318,251.099579228695));
#22821=CARTESIAN_POINT('Ctrl Pts',(253.152688209842,184.229566394342,251.219678850939));
#22822=CARTESIAN_POINT('Ctrl Pts',(253.071947254646,184.323639013818,251.342475391721));
#22823=CARTESIAN_POINT('Ctrl Pts',(252.993394165095,184.416208073786,251.467962021102));
#22824=CARTESIAN_POINT('Ctrl Pts',(252.945942178244,184.47212676319,251.543765403519));
#22825=CARTESIAN_POINT('Ctrl Pts',(252.899289102358,184.527496308855,251.620551219808));
#22826=CARTESIAN_POINT('Ctrl Pts',(252.853402096841,184.582281191483,251.698323923814));
#22827=CARTESIAN_POINT('Ctrl Pts',(252.792477402011,184.655019698123,251.8015836202));
#22828=CARTESIAN_POINT('Ctrl Pts',(252.732831847409,184.726825457145,251.906717635845));
#22829=CARTESIAN_POINT('Ctrl Pts',(252.674625268463,184.797384011339,252.013355098741));
#22830=CARTESIAN_POINT('Ctrl Pts',(252.616418689517,184.867942565532,252.119992561637));
#22831=CARTESIAN_POINT('Ctrl Pts',(252.559651171105,184.937253744578,252.228133237983));
#22832=CARTESIAN_POINT('Ctrl Pts',(252.504457767201,185.005044677865,252.337370321838));
#22833=CARTESIAN_POINT('Ctrl Pts',(252.42657046849,185.100709237347,252.491522462831));
#22834=CARTESIAN_POINT('Ctrl Pts',(252.351675222557,185.193488613487,252.648102763049));
#22835=CARTESIAN_POINT('Ctrl Pts',(252.279627173469,185.283369929189,252.8070552405));
#22836=CARTESIAN_POINT('Ctrl Pts',(252.205887223038,185.375361924093,252.969740392375));
#22837=CARTESIAN_POINT('Ctrl Pts',(252.135129557654,185.464318441126,253.134910972967));
#22838=CARTESIAN_POINT('Ctrl Pts',(252.067226908187,185.550195451901,253.302543574781));
#22839=CARTESIAN_POINT('Ctrl Pts',(252.013418480972,185.618247389785,253.435381493836));
#22840=CARTESIAN_POINT('Ctrl Pts',(251.961403419595,185.684364966429,253.569766278894));
#22841=CARTESIAN_POINT('Ctrl Pts',(251.911131498665,185.748511641906,253.705698605741));
#22842=CARTESIAN_POINT('Ctrl Pts',(251.845227331299,185.83260497191,253.883899610465));
#22843=CARTESIAN_POINT('Ctrl Pts',(251.782324757381,185.913318714639,254.064750713446));
#22844=CARTESIAN_POINT('Ctrl Pts',(251.722366218587,185.99060689966,254.248259140579));
#22845=CARTESIAN_POINT('Ctrl Pts',(251.662264405385,186.068079769288,254.432206071753));
#22846=CARTESIAN_POINT('Ctrl Pts',(251.605120605634,186.142110878666,254.618823595358));
#22847=CARTESIAN_POINT('Ctrl Pts',(251.550905771698,186.212615651627,254.808139774963));
#22848=CARTESIAN_POINT('Ctrl Pts',(251.515017728347,186.259286980575,254.933459484857));
#22849=CARTESIAN_POINT('Ctrl Pts',(251.480413730466,186.304412307625,255.059962134081));
#22850=CARTESIAN_POINT('Ctrl Pts',(251.447092607203,186.347957341824,255.187659050152));
#22851=CARTESIAN_POINT('Ctrl Pts',(251.413623787562,186.391695390037,255.31592198471));
#22852=CARTESIAN_POINT('Ctrl Pts',(251.381388138616,186.433927793499,255.445645779032));
#22853=CARTESIAN_POINT('Ctrl Pts',(251.350508544363,186.47446346869,255.576380416569));
#22854=CARTESIAN_POINT('Ctrl Pts',(251.321175965177,186.512968375609,255.70056547148));
#22855=CARTESIAN_POINT('Ctrl Pts',(251.293066796372,186.549942577642,255.825662190079));
#22856=CARTESIAN_POINT('Ctrl Pts',(251.266260224554,186.585265045835,255.951266227758));
#22857=CARTESIAN_POINT('Ctrl Pts',(251.264846432393,186.587127970679,255.957890648253));
#22858=CARTESIAN_POINT('Ctrl Pts',(251.263436257508,186.588986310925,255.964516476233));
#22859=CARTESIAN_POINT('Ctrl Pts',(251.262029709513,186.590840052102,255.971143651196));
#22860=CARTESIAN_POINT('Ctrl Pts',(251.22001307173,186.646215319669,256.169111734006));
#22861=CARTESIAN_POINT('Ctrl Pts',(251.181280148853,186.697414865585,256.36803659797));
#22862=CARTESIAN_POINT('Ctrl Pts',(251.14573394388,186.744500799677,256.567896415216));
#22863=CARTESIAN_POINT('Ctrl Pts',(251.133775781622,186.760341062803,256.635131613045));
#22864=CARTESIAN_POINT('Ctrl Pts',(251.122178501551,186.775715462994,256.702472823652));
#22865=CARTESIAN_POINT('Ctrl Pts',(251.110939119017,186.790625402752,256.769919772245));
#22866=CARTESIAN_POINT('Ctrl Pts',(251.07666058089,186.83609862487,256.975623492344));
#22867=CARTESIAN_POINT('Ctrl Pts',(251.045703415176,186.877231614162,257.182305293813));
#22868=CARTESIAN_POINT('Ctrl Pts',(251.01801554753,186.914072166413,257.389953006453));
#22869=CARTESIAN_POINT('Ctrl Pts',(250.988873109874,186.952848120953,257.608509400803));
#22870=CARTESIAN_POINT('Ctrl Pts',(250.963352139096,186.986869307684,257.828136343562));
#22871=CARTESIAN_POINT('Ctrl Pts',(250.941425713081,187.016143062935,258.048838461296));
#22872=CARTESIAN_POINT('Ctrl Pts',(250.92055028519,187.044013640948,258.258961677032));
#22873=CARTESIAN_POINT('Ctrl Pts',(250.902933271537,187.067580711243,258.470060113447));
#22874=CARTESIAN_POINT('Ctrl Pts',(250.888581473397,187.086807478048,258.682145548763));
#22875=CARTESIAN_POINT('Ctrl Pts',(250.874282432124,187.105963567715,258.893451363066));
#22876=CARTESIAN_POINT('Ctrl Pts',(250.863224638294,187.120811223589,259.105737473469));
#22877=CARTESIAN_POINT('Ctrl Pts',(250.855444255506,187.131271651202,259.319014860937));
#22878=CARTESIAN_POINT('Ctrl Pts',(250.847728740891,187.141644866032,259.530514069237));
#22879=CARTESIAN_POINT('Ctrl Pts',(250.843236249268,187.14770366393,259.742988617007));
#22880=CARTESIAN_POINT('Ctrl Pts',(250.842030805421,187.149329638876,259.956440655387));
#22881=CARTESIAN_POINT('Ctrl Pts',(250.841827424176,187.149603971695,259.992454063485));
#22882=CARTESIAN_POINT('Ctrl Pts',(250.841717678375,187.149752023718,260.02849526646));
#22883=CARTESIAN_POINT('Ctrl Pts',(250.841701955889,187.149773109793,260.06456423381));
#22884=CARTESIAN_POINT('Ctrl Pts',(250.841606110561,187.149901651909,260.284443062896));
#22885=CARTESIAN_POINT('Ctrl Pts',(250.845007611412,187.145332323719,260.503797799271));
#22886=CARTESIAN_POINT('Ctrl Pts',(250.851874504217,187.136124450971,260.722610014815));
#22887=CARTESIAN_POINT('Ctrl Pts',(250.858758705094,187.126893369687,260.941973748737));
#22888=CARTESIAN_POINT('Ctrl Pts',(250.869125789004,187.113000327815,261.160792798172));
#22889=CARTESIAN_POINT('Ctrl Pts',(250.882973567754,187.094462308955,261.379050191942));
#22890=CARTESIAN_POINT('Ctrl Pts',(250.890649367219,187.084186717624,261.500029882383));
#22891=CARTESIAN_POINT('Ctrl Pts',(250.899395130637,187.072483214165,261.620836984648));
#22892=CARTESIAN_POINT('Ctrl Pts',(250.909214425574,187.059349078077,261.74146783121));
#22893=CARTESIAN_POINT('Ctrl Pts',(250.92293432421,187.040997555189,261.910017915268));
#22894=CARTESIAN_POINT('Ctrl Pts',(250.938765555668,187.019841072376,262.078357348699));
#22895=CARTESIAN_POINT('Ctrl Pts',(250.956686462005,186.995918549522,262.246081476918));
#22896=CARTESIAN_POINT('Ctrl Pts',(250.974606765734,186.971996831088,262.413799965246));
#22897=CARTESIAN_POINT('Ctrl Pts',(250.994616582585,186.945309301798,262.580902869183));
#22898=CARTESIAN_POINT('Ctrl Pts',(251.016668245256,186.915939341316,262.746993592085));
#22899=CARTESIAN_POINT('Ctrl Pts',(251.03875414947,186.88652377553,262.913342218557));
#22900=CARTESIAN_POINT('Ctrl Pts',(251.062888205982,186.854417515176,263.078675204227));
#22901=CARTESIAN_POINT('Ctrl Pts',(251.088996878786,186.819748071741,263.242606920757));
#22902=CARTESIAN_POINT('Ctrl Pts',(251.096643466719,186.809594244704,263.290618487446));
#22903=CARTESIAN_POINT('Ctrl Pts',(251.104459264335,186.799220839185,263.338509959372));
#22904=CARTESIAN_POINT('Ctrl Pts',(251.112442017969,186.788631750385,263.386271915724));
#22905=CARTESIAN_POINT('Ctrl Pts',(251.146825606285,186.743022066478,263.59199384073));
#22906=CARTESIAN_POINT('Ctrl Pts',(251.184376063794,186.693300712314,263.795768788702));
#22907=CARTESIAN_POINT('Ctrl Pts',(251.225096534777,186.639543062093,263.997613250195));
#22908=CARTESIAN_POINT('Ctrl Pts',(251.265759643961,186.585861138784,264.199173378989));
#22909=CARTESIAN_POINT('Ctrl Pts',(251.309583903252,186.528154160268,264.398809008199));
#22910=CARTESIAN_POINT('Ctrl Pts',(251.356601925706,186.466456182231,264.596524895168));
#22911=CARTESIAN_POINT('Ctrl Pts',(251.385290342217,186.428810675265,264.717162799956));
#22912=CARTESIAN_POINT('Ctrl Pts',(251.415168345009,186.389678556072,264.837085736718));
#22913=CARTESIAN_POINT('Ctrl Pts',(251.446248574714,186.349060370531,264.956291312693));
#22914=CARTESIAN_POINT('Ctrl Pts',(251.507611543227,186.268866225762,265.191643756174));
#22915=CARTESIAN_POINT('Ctrl Pts',(251.573766438657,186.182742940431,265.424589848528));
#22916=CARTESIAN_POINT('Ctrl Pts',(251.64473576945,186.090888515716,265.65451838021));
#22917=CARTESIAN_POINT('Ctrl Pts',(251.716280282574,185.998289642073,265.886310404581));
#22918=CARTESIAN_POINT('Ctrl Pts',(251.792717524411,185.899866376696,266.115035751658));
#22919=CARTESIAN_POINT('Ctrl Pts',(251.874053462935,185.795871094589,266.340075157387));
#22920=CARTESIAN_POINT('Ctrl Pts',(251.886945199337,185.779387854975,266.375743875929));
#22921=CARTESIAN_POINT('Ctrl Pts',(251.899959968139,185.762764733898,266.411320009294));
#22922=CARTESIAN_POINT('Ctrl Pts',(251.913097755267,185.746002848768,266.44680110693));
#22923=CARTESIAN_POINT('Ctrl Pts',(251.977474654705,185.663867388441,266.620663191333));
#22924=CARTESIAN_POINT('Ctrl Pts',(252.044458836526,185.578824893745,266.791326093399));
#22925=CARTESIAN_POINT('Ctrl Pts',(252.114089196345,185.491018016114,266.958844062153));
#22926=CARTESIAN_POINT('Ctrl Pts',(252.183213825263,185.403848886895,267.125145334431));
#22927=CARTESIAN_POINT('Ctrl Pts',(252.254946455527,185.313955174931,267.288347764576));
#22928=CARTESIAN_POINT('Ctrl Pts',(252.329354941905,185.221440043281,267.448484623448));
#22929=CARTESIAN_POINT('Ctrl Pts',(252.387524576895,185.14911534349,267.573673336223));
#22930=CARTESIAN_POINT('Ctrl Pts',(252.447330174334,185.075187810648,267.696988229989));
#22931=CARTESIAN_POINT('Ctrl Pts',(252.508816167603,184.999692362965,267.818433227061));
#22932=CARTESIAN_POINT('Ctrl Pts',(252.581135618947,184.91089507654,267.961276094028));
#22933=CARTESIAN_POINT('Ctrl Pts',(252.655762335573,184.819908038571,268.101520561569));
#22934=CARTESIAN_POINT('Ctrl Pts',(252.732846686904,184.726874324985,268.239179237566));
#22935=CARTESIAN_POINT('Ctrl Pts',(252.811212430181,184.63229408932,268.379126247261));
#22936=CARTESIAN_POINT('Ctrl Pts',(252.892118157875,184.535598533268,268.516401736792));
#22937=CARTESIAN_POINT('Ctrl Pts',(252.975755262267,184.436907602098,268.650984600091));
#22938=CARTESIAN_POINT('Ctrl Pts',(253.05354173932,184.345120351587,268.77615305115));
#22939=CARTESIAN_POINT('Ctrl Pts',(253.133691256943,184.251606716133,268.898992714716));
#22940=CARTESIAN_POINT('Ctrl Pts',(253.216382790853,184.156441034041,269.019449088555));
#22941=CARTESIAN_POINT('Ctrl Pts',(253.222602346838,184.149283248235,269.028509086906));
#22942=CARTESIAN_POINT('Ctrl Pts',(253.228836294106,184.142116107116,269.037555582614));
#22943=CARTESIAN_POINT('Ctrl Pts',(253.23508471398,184.134939637759,269.046588542386));
#22944=CARTESIAN_POINT('Ctrl Pts',(253.306413051232,184.053017225876,269.149703572094));
#22945=CARTESIAN_POINT('Ctrl Pts',(253.379751629605,183.969770389543,269.251215988406));
#22946=CARTESIAN_POINT('Ctrl Pts',(253.455018913012,183.885679746065,269.350694801928));
#22947=CARTESIAN_POINT('Ctrl Pts',(253.520365632475,183.812672624774,269.437061863759));
#22948=CARTESIAN_POINT('Ctrl Pts',(253.587165865471,183.739030223278,269.521896731626));
#22949=CARTESIAN_POINT('Ctrl Pts',(253.655357308654,183.66508985876,269.604937666439));
#22950=CARTESIAN_POINT('Ctrl Pts',(253.721469993782,183.593403503266,269.685447169095));
#22951=CARTESIAN_POINT('Ctrl Pts',(253.788913289867,183.521349913543,269.764328269069));
#22952=CARTESIAN_POINT('Ctrl Pts',(253.857933938861,183.449186383109,269.841586336771));
#22953=CARTESIAN_POINT('Ctrl Pts',(253.923031167831,183.381124927118,269.914452735395));
#22954=CARTESIAN_POINT('Ctrl Pts',(253.989531816038,183.312965555382,269.985875904148));
#22955=CARTESIAN_POINT('Ctrl Pts',(254.057666508963,183.244906879936,270.05582404412));
#22956=CARTESIAN_POINT('Ctrl Pts',(254.077627986578,183.224967673225,270.076316808823));
#22957=CARTESIAN_POINT('Ctrl Pts',(254.097729863561,183.205036996922,270.096682691231));
#22958=CARTESIAN_POINT('Ctrl Pts',(254.117978295483,183.185119561377,270.116920145927));
#22959=CARTESIAN_POINT('Ctrl Pts',(254.168638618129,183.135287371168,270.167553004235));
#22960=CARTESIAN_POINT('Ctrl Pts',(254.220156691413,183.085397762633,270.217392754447));
#22961=CARTESIAN_POINT('Ctrl Pts',(254.272829857711,183.035824074896,270.266425929164));
#22962=CARTESIAN_POINT('Ctrl Pts',(254.322838834282,182.988757806381,270.312979023613));
#22963=CARTESIAN_POINT('Ctrl Pts',(254.373889180299,182.941976341435,270.358805695447));
#22964=CARTESIAN_POINT('Ctrl Pts',(254.426257942816,182.895783796577,270.403857842544));
#22965=CARTESIAN_POINT('Ctrl Pts',(254.474749681505,182.853011030771,270.445574637814));
#22966=CARTESIAN_POINT('Ctrl Pts',(254.524372093986,182.810743225032,270.486627733615));
#22967=CARTESIAN_POINT('Ctrl Pts',(254.575362051097,182.769208050738,270.526939979175));
#22968=CARTESIAN_POINT('Ctrl Pts',(254.597512071361,182.751165184957,270.544451605123));
#22969=CARTESIAN_POINT('Ctrl Pts',(254.619920357463,182.733260383457,270.561822875596));
#22970=CARTESIAN_POINT('Ctrl Pts',(254.642607244695,182.715511376955,270.57904459608));
#22971=CARTESIAN_POINT('Ctrl Pts',(254.677375991624,182.688310169977,270.605437711852));
#22972=CARTESIAN_POINT('Ctrl Pts',(254.712661735147,182.661478290065,270.6314136033));
#22973=CARTESIAN_POINT('Ctrl Pts',(254.74879651668,182.635472037571,270.656922763078));
#22974=CARTESIAN_POINT('Ctrl Pts',(254.781575063799,182.611881271649,270.680062606749));
#22975=CARTESIAN_POINT('Ctrl Pts',(254.815052444963,182.588969919988,270.702818651702));
#22976=CARTESIAN_POINT('Ctrl Pts',(254.849491525827,182.56706552931,270.725118538041));
#22977=CARTESIAN_POINT('Ctrl Pts',(254.881214538541,182.546888647507,270.745659724394));
#22978=CARTESIAN_POINT('Ctrl Pts',(254.913753677733,182.52756625059,270.765814146755));
#22979=CARTESIAN_POINT('Ctrl Pts',(254.947325690666,182.509341768866,270.785489860278));
#22980=CARTESIAN_POINT('Ctrl Pts',(254.974874835784,182.494386785597,270.801635722257));
#22981=CARTESIAN_POINT('Ctrl Pts',(255.003234322111,182.480064149302,270.817544015284));
#22982=CARTESIAN_POINT('Ctrl Pts',(255.032557552846,182.467371520176,270.832831465269));
#22983=CARTESIAN_POINT('Ctrl Pts',(255.057876881517,182.456411989439,270.846031510456));
#22984=CARTESIAN_POINT('Ctrl Pts',(255.083914893497,182.446667929592,270.858769003089));
#22985=CARTESIAN_POINT('Ctrl Pts',(255.110781390828,182.438767974361,270.870757623905));
#22986=CARTESIAN_POINT('Ctrl Pts',(255.115029956242,182.437518705572,270.872653458674));
#22987=CARTESIAN_POINT('Ctrl Pts',(255.119299262443,182.436315516993,270.874530468985));
#22988=CARTESIAN_POINT('Ctrl Pts',(255.123589769808,182.435160851133,270.876387405171));
#22989=CARTESIAN_POINT('Ctrl Pts',(255.145641523356,182.429226259998,270.885931427743));
#22990=CARTESIAN_POINT('Ctrl Pts',(255.168614853771,182.424524354017,270.895088038127));
#22991=CARTESIAN_POINT('Ctrl Pts',(255.192182661757,182.42240360197,270.90314026354));
#22992=CARTESIAN_POINT('Ctrl Pts',(255.202197358502,182.421502428274,270.906561905285));
#22993=CARTESIAN_POINT('Ctrl Pts',(255.212319486848,182.421067151468,270.909783638002));
#22994=CARTESIAN_POINT('Ctrl Pts',(255.222524416932,182.421200143345,270.912747626903));
#22995=CARTESIAN_POINT('Ctrl Pts',(255.241300295314,182.421444832853,270.918201019985));
#22996=CARTESIAN_POINT('Ctrl Pts',(255.260574263975,182.423855159518,270.922749881881));
#22997=CARTESIAN_POINT('Ctrl Pts',(255.27922678993,182.429091333001,270.925735589379));
#22998=CARTESIAN_POINT('Ctrl Pts',(255.294569863377,182.433398470518,270.928191553227));
#22999=CARTESIAN_POINT('Ctrl Pts',(255.309492000005,182.439617991123,270.929590730021));
#23000=CARTESIAN_POINT('Ctrl Pts',(255.323361884753,182.448125072317,270.929590730047));
#23001=CARTESIAN_POINT('Ctrl Pts',(255.69795971203,182.760768310083,270.863289666853));
#23002=CARTESIAN_POINT('Ctrl Pts',(255.542065616723,182.787419934355,270.793196892032));
#23003=CARTESIAN_POINT('Ctrl Pts',(255.379913538211,182.835032555837,270.757496758746));
#23004=CARTESIAN_POINT('Ctrl Pts',(255.788387377274,182.6113076933,270.977299065995));
#23005=CARTESIAN_POINT('Ctrl Pts',(255.630549472211,182.637016714706,270.909459407662));
#23006=CARTESIAN_POINT('Ctrl Pts',(255.466168344799,182.672413168797,270.864172365102));
#23007=CARTESIAN_POINT('Ctrl Pts',(255.619077812391,182.348069925451,271.063276557297));
#23008=CARTESIAN_POINT('Ctrl Pts',(255.520634101689,182.412422779613,270.996082559504));
#23009=CARTESIAN_POINT('Ctrl Pts',(255.41911229268,182.482769694297,270.941201198992));
#23010=CARTESIAN_POINT('Ctrl Pts',(255.309081965699,182.194018031453,271.043748001287));
#23011=CARTESIAN_POINT('Ctrl Pts',(255.284781185601,182.30336100112,270.976399337839));
#23012=CARTESIAN_POINT('Ctrl Pts',(255.256048943706,182.419383189339,270.923589021742));
#23013=CARTESIAN_POINT('Ctrl Pts',(255.227638836467,182.171517318723,271.028894764525));
#23014=CARTESIAN_POINT('Ctrl Pts',(255.220900220453,182.291278840731,270.961419415091));
#23015=CARTESIAN_POINT('Ctrl Pts',(255.209076752236,182.418439019625,270.910193902727));
#23016=CARTESIAN_POINT('Ctrl Pts',(254.992369492328,182.139063052789,270.967594315179));
#23017=CARTESIAN_POINT('Ctrl Pts',(255.033034731904,182.286438498041,270.89962152934));
#23018=CARTESIAN_POINT('Ctrl Pts',(255.065868025329,182.444215095646,270.85481550798));
#23019=CARTESIAN_POINT('Ctrl Pts',(254.845276603423,182.158294666748,270.906629200941));
#23020=CARTESIAN_POINT('Ctrl Pts',(254.911582333463,182.319980569757,270.838166406986));
#23021=CARTESIAN_POINT('Ctrl Pts',(254.967189227365,182.494967621995,270.79962270377));
#23022=CARTESIAN_POINT('Ctrl Pts',(254.575314234875,182.219156544986,270.776054410111));
#23023=CARTESIAN_POINT('Ctrl Pts',(254.686367581278,182.40516109745,270.706733188276));
#23024=CARTESIAN_POINT('Ctrl Pts',(254.779991222184,182.61080632492,270.680873498225));
#23025=CARTESIAN_POINT('Ctrl Pts',(254.449480404597,182.262946994164,270.704357325665));
#23026=CARTESIAN_POINT('Ctrl Pts',(254.579931124656,182.459173024266,270.634591588456));
#23027=CARTESIAN_POINT('Ctrl Pts',(254.689080556251,182.678457051227,270.61544244106));
#23028=CARTESIAN_POINT('Ctrl Pts',(254.208537366376,182.362149671029,270.552986112183));
#23029=CARTESIAN_POINT('Ctrl Pts',(254.374787969265,182.57680023898,270.48243337455));
#23030=CARTESIAN_POINT('Ctrl Pts',(254.511233959241,182.821808313659,270.476716822089));
#23031=CARTESIAN_POINT('Ctrl Pts',(254.095280913377,182.417198764343,270.474272667784));
#23032=CARTESIAN_POINT('Ctrl Pts',(254.277625278501,182.63991040501,270.403355923987));
#23033=CARTESIAN_POINT('Ctrl Pts',(254.425574355397,182.896754769307,270.404307171622));
#23034=CARTESIAN_POINT('Ctrl Pts',(253.769243527662,182.59039034952,270.230560291979));
#23035=CARTESIAN_POINT('Ctrl Pts',(253.996372167823,182.835464225051,270.158425854918));
#23036=CARTESIAN_POINT('Ctrl Pts',(254.175230499608,183.125969043173,270.179232040224));
#23037=CARTESIAN_POINT('Ctrl Pts',(253.570030440553,182.716405639144,270.058020584565));
#23038=CARTESIAN_POINT('Ctrl Pts',(253.823130620869,182.973594173456,269.985397145909));
#23039=CARTESIAN_POINT('Ctrl Pts',(254.017113051129,183.284502373521,270.018746187404));
#23040=CARTESIAN_POINT('Ctrl Pts',(253.193152505323,182.973731799716,269.695353089176));
#23041=CARTESIAN_POINT('Ctrl Pts',(253.494005385797,183.252498852315,269.622233265112));
#23042=CARTESIAN_POINT('Ctrl Pts',(253.712692616096,183.602487682801,269.678924564811));
#23043=CARTESIAN_POINT('Ctrl Pts',(253.015610508868,183.10569901033,269.504802628584));
#23044=CARTESIAN_POINT('Ctrl Pts',(253.338259190744,183.393881117277,269.43160775279));
#23045=CARTESIAN_POINT('Ctrl Pts',(253.566313219562,183.76249158633,269.499192996309));
#23046=CARTESIAN_POINT('Ctrl Pts',(252.510219054762,183.500014386828,268.90971068143));
#23047=CARTESIAN_POINT('Ctrl Pts',(252.892708926363,183.814710175669,268.835653720007));
#23048=CARTESIAN_POINT('Ctrl Pts',(253.144000705384,184.236445869242,268.934147470799));
#23049=CARTESIAN_POINT('Ctrl Pts',(252.21379797866,183.756625851448,268.487768626105));
#23050=CARTESIAN_POINT('Ctrl Pts',(252.630928206058,184.084365475791,268.414865728006));
#23051=CARTESIAN_POINT('Ctrl Pts',(252.888614147946,184.539611307648,268.528724253357));
#23052=CARTESIAN_POINT('Ctrl Pts',(251.678465949766,184.239590353276,267.596296773091));
#23053=CARTESIAN_POINT('Ctrl Pts',(252.156838953501,184.590134712182,267.527194887727));
#23054=CARTESIAN_POINT('Ctrl Pts',(252.420283367909,185.108451280444,267.662745539141));
#23055=CARTESIAN_POINT('Ctrl Pts',(251.440149873111,184.466440448225,267.126721548513));
#23056=CARTESIAN_POINT('Ctrl Pts',(251.945666293451,184.826117950235,267.060380338219));
#23057=CARTESIAN_POINT('Ctrl Pts',(252.207603382145,185.374426340438,267.202149362294));
#23058=CARTESIAN_POINT('Ctrl Pts',(251.120880433865,184.778331207481,266.386173310803));
#23059=CARTESIAN_POINT('Ctrl Pts',(251.662713290358,185.149605958963,266.32613025419));
#23060=CARTESIAN_POINT('Ctrl Pts',(251.919413580121,185.740053888074,266.46935921003));
#23061=CARTESIAN_POINT('Ctrl Pts',(251.020631854738,184.877861632215,266.132433857755));
#23062=CARTESIAN_POINT('Ctrl Pts',(251.573717325274,185.252826583724,266.074271837757));
#23063=CARTESIAN_POINT('Ctrl Pts',(251.828285193104,185.856697231355,266.217256414804));
#23064=CARTESIAN_POINT('Ctrl Pts',(250.835058673596,185.064199897975,265.619443034692));
#23065=CARTESIAN_POINT('Ctrl Pts',(251.408881398008,185.445954511362,265.56525067354));
#23066=CARTESIAN_POINT('Ctrl Pts',(251.658709051878,186.075107733935,265.705670744697));
#23067=CARTESIAN_POINT('Ctrl Pts',(250.749449478807,185.151281700865,265.359658969482));
#23068=CARTESIAN_POINT('Ctrl Pts',(251.332858495523,185.536071698513,265.307631788323));
#23069=CARTESIAN_POINT('Ctrl Pts',(251.580006721225,186.177194952975,265.445667169421));
#23070=CARTESIAN_POINT('Ctrl Pts',(250.512931393725,185.393971069805,264.570646581531));
#23071=CARTESIAN_POINT('Ctrl Pts',(251.122429833441,185.787492196982,264.524265624361));
#23072=CARTESIAN_POINT('Ctrl Pts',(251.361638634229,186.461806439964,264.653490036942));
#23073=CARTESIAN_POINT('Ctrl Pts',(250.382202619427,185.531072224838,264.031800236087));
#23074=CARTESIAN_POINT('Ctrl Pts',(251.006472559572,185.928841924294,263.990771434713));
#23075=CARTESIAN_POINT('Ctrl Pts',(251.239619961047,186.622748967039,264.109175603941));
#23076=CARTESIAN_POINT('Ctrl Pts',(250.171863847949,185.753517650536,262.928444837571));
#23077=CARTESIAN_POINT('Ctrl Pts',(250.819578279876,186.158438332912,262.898037648395));
#23078=CARTESIAN_POINT('Ctrl Pts',(251.042392746885,186.884097112,262.989762845941));
#23079=CARTESIAN_POINT('Ctrl Pts',(250.092065247842,185.839108858332,262.360616500679));
#23080=CARTESIAN_POINT('Ctrl Pts',(250.748811398794,186.246530121276,262.336402006455));
#23081=CARTESIAN_POINT('Ctrl Pts',(250.966993715978,186.984782734557,262.411264016072));
#23082=CARTESIAN_POINT('Ctrl Pts',(249.986394459609,185.952757018574,261.21805700291));
#23083=CARTESIAN_POINT('Ctrl Pts',(250.654929677702,186.363693623886,261.205549911323));
#23084=CARTESIAN_POINT('Ctrl Pts',(250.86699061522,187.118523637578,261.244648862485));
#23085=CARTESIAN_POINT('Ctrl Pts',(249.960109375638,185.981256709722,260.643179975231));
#23086=CARTESIAN_POINT('Ctrl Pts',(250.631625253859,186.393001588752,260.637234645382));
#23087=CARTESIAN_POINT('Ctrl Pts',(250.842000505805,187.152093026429,260.656413628318));
#23088=CARTESIAN_POINT('Ctrl Pts',(249.960905241707,185.980396154132,258.908570805387));
#23089=CARTESIAN_POINT('Ctrl Pts',(250.632332281791,186.392114734583,258.920748434052));
#23090=CARTESIAN_POINT('Ctrl Pts',(250.84275598636,187.151079700571,258.881502896051));
#23091=CARTESIAN_POINT('Ctrl Pts',(250.065633252246,185.865882874739,257.778333653513));
#23092=CARTESIAN_POINT('Ctrl Pts',(250.724653494205,186.275071296267,257.806485704709));
#23093=CARTESIAN_POINT('Ctrl Pts',(250.942775774683,187.016113768484,257.725189584552));
#23094=CARTESIAN_POINT('Ctrl Pts',(250.380864499977,185.532477343041,256.121241766934));
#23095=CARTESIAN_POINT('Ctrl Pts',(251.00528385278,185.93029262334,256.162216522362));
#23096=CARTESIAN_POINT('Ctrl Pts',(251.238370010026,186.624398843282,256.043933065562));
#23097=CARTESIAN_POINT('Ctrl Pts',(250.514011721928,185.392842215478,255.57225813953));
#23098=CARTESIAN_POINT('Ctrl Pts',(251.123387551199,185.786328698607,255.618684551377));
#23099=CARTESIAN_POINT('Ctrl Pts',(251.362645044373,186.460481651283,255.489375917092));
#23100=CARTESIAN_POINT('Ctrl Pts',(250.830318559901,185.068323104174,254.518436453205));
#23101=CARTESIAN_POINT('Ctrl Pts',(251.404418795496,185.45059063801,254.573829497636));
#23102=CARTESIAN_POINT('Ctrl Pts',(251.654661916545,186.07990581835,254.431367315278));
#23103=CARTESIAN_POINT('Ctrl Pts',(251.01372557053,184.883066549833,254.010308997639));
#23104=CARTESIAN_POINT('Ctrl Pts',(251.567097640648,185.258971787377,254.069913461328));
#23105=CARTESIAN_POINT('Ctrl Pts',(251.82266868169,185.862831131789,253.92454353509));
#23106=CARTESIAN_POINT('Ctrl Pts',(251.435183105815,184.471236242898,253.031245832271));
#23107=CARTESIAN_POINT('Ctrl Pts',(251.941270764064,184.8310916679,253.097487852073));
#23108=CARTESIAN_POINT('Ctrl Pts',(252.203142475808,185.380049794653,252.955669568942));
#23109=CARTESIAN_POINT('Ctrl Pts',(251.673063255092,184.244533938978,252.560299088865));
#23110=CARTESIAN_POINT('Ctrl Pts',(252.152028447736,184.595329145257,252.629402359262));
#23111=CARTESIAN_POINT('Ctrl Pts',(252.415532683477,185.114266209537,252.493606043876));
#23112=CARTESIAN_POINT('Ctrl Pts',(252.214767072122,183.755682726479,251.65739454731));
#23113=CARTESIAN_POINT('Ctrl Pts',(252.631765976759,184.083410260715,251.730354544452));
#23114=CARTESIAN_POINT('Ctrl Pts',(252.88948604426,184.538507962755,251.616471964354));
#23115=CARTESIAN_POINT('Ctrl Pts',(252.513395480913,183.497442401041,251.233479557366));
#23116=CARTESIAN_POINT('Ctrl Pts',(252.895520198024,183.811972357617,251.307525668854));
#23117=CARTESIAN_POINT('Ctrl Pts',(253.146682958596,184.23337465506,251.209228221821));
#23118=CARTESIAN_POINT('Ctrl Pts',(253.016637605481,183.104944858353,250.641303159677));
#23119=CARTESIAN_POINT('Ctrl Pts',(253.339162767622,183.393068983501,250.714493355331));
#23120=CARTESIAN_POINT('Ctrl Pts',(253.567157366365,183.761574936337,250.646975576108));
#23121=CARTESIAN_POINT('Ctrl Pts',(253.193960610691,182.973101659209,250.450914901744));
#23122=CARTESIAN_POINT('Ctrl Pts',(253.494711976584,183.251831639529,250.524039761223));
#23123=CARTESIAN_POINT('Ctrl Pts',(253.713366926182,183.601731584937,250.467392937178));
#23124=CARTESIAN_POINT('Ctrl Pts',(253.573217473954,182.714308793454,250.086240949678));
#23125=CARTESIAN_POINT('Ctrl Pts',(253.825903660531,182.971313112234,250.158863657386));
#23126=CARTESIAN_POINT('Ctrl Pts',(254.019665577714,183.281888396407,250.125707988976));
#23127=CARTESIAN_POINT('Ctrl Pts',(253.773477418047,182.587816240006,249.913093051726));
#23128=CARTESIAN_POINT('Ctrl Pts',(254.0000449561,182.832626574658,249.985218181233));
#23129=CARTESIAN_POINT('Ctrl Pts',(254.178563913084,183.122695807423,249.964674450387));
#23130=CARTESIAN_POINT('Ctrl Pts',(254.100587499649,182.414548019999,249.669137321989));
#23131=CARTESIAN_POINT('Ctrl Pts',(254.282183330116,182.63688758736,249.740038146342));
#23132=CARTESIAN_POINT('Ctrl Pts',(254.429606317529,182.893177505095,249.739400387974));
#23133=CARTESIAN_POINT('Ctrl Pts',(254.214569077146,182.359411089098,249.590185103147));
#23134=CARTESIAN_POINT('Ctrl Pts',(254.379947576733,182.573617767892,249.660717158142));
#23135=CARTESIAN_POINT('Ctrl Pts',(254.515748475552,182.817990681841,249.66678196835));
#23136=CARTESIAN_POINT('Ctrl Pts',(254.454267136741,182.261243106653,249.440057780993));
#23137=CARTESIAN_POINT('Ctrl Pts',(254.583984420675,182.457082712603,249.509806195947));
#23138=CARTESIAN_POINT('Ctrl Pts',(254.69254854312,182.675848723747,249.529212381473));
#23139=CARTESIAN_POINT('Ctrl Pts',(254.579431140785,182.217862721287,249.368887742416));
#23140=CARTESIAN_POINT('Ctrl Pts',(254.689836547022,182.403523225518,249.438195157897));
#23141=CARTESIAN_POINT('Ctrl Pts',(254.782932458239,182.608716259834,249.464266972048));
#23142=CARTESIAN_POINT('Ctrl Pts',(254.850321649343,182.157535534843,249.238378443436));
#23143=CARTESIAN_POINT('Ctrl Pts',(254.915754746099,182.318738837607,249.306825880349));
#23144=CARTESIAN_POINT('Ctrl Pts',(254.970598124639,182.493137486537,249.345587340743));
#23145=CARTESIAN_POINT('Ctrl Pts',(254.998038973668,182.139292856471,249.177802136601));
#23146=CARTESIAN_POINT('Ctrl Pts',(255.037620113726,182.286044696427,249.245759936704));
#23147=CARTESIAN_POINT('Ctrl Pts',(255.069446631777,182.443110220345,249.290752656895));
#23148=CARTESIAN_POINT('Ctrl Pts',(255.229449025207,182.172051550256,249.117980902794));
#23149=CARTESIAN_POINT('Ctrl Pts',(255.222316999038,182.291578833741,249.185453386513));
#23150=CARTESIAN_POINT('Ctrl Pts',(255.210112882693,182.418489907288,249.236712388294));
#23151=CARTESIAN_POINT('Ctrl Pts',(255.309938799049,182.194435982025,249.103380034896));
#23152=CARTESIAN_POINT('Ctrl Pts',(255.28543412136,182.303655305446,249.17072821894));
#23153=CARTESIAN_POINT('Ctrl Pts',(255.25650145862,182.41955152691,249.223544729758));
#23154=CARTESIAN_POINT('Ctrl Pts',(255.616775680461,182.346950242796,249.084067933231));
#23155=CARTESIAN_POINT('Ctrl Pts',(255.518880630488,182.411635590028,249.151263131289));
#23156=CARTESIAN_POINT('Ctrl Pts',(255.417895727355,182.482320258294,249.206127762022));
#23157=CARTESIAN_POINT('Ctrl Pts',(255.791381968628,182.610038677597,249.16820680786));
#23158=CARTESIAN_POINT('Ctrl Pts',(255.633022052011,182.635401590256,249.235995576485));
#23159=CARTESIAN_POINT('Ctrl Pts',(255.468204518472,182.670314620703,249.281404339452));
#23160=CARTESIAN_POINT('Ctrl Pts',(255.694913445605,182.768215148388,249.288918868784));
#23161=CARTESIAN_POINT('Ctrl Pts',(255.539407953281,182.795436716082,249.359305602731));
#23162=CARTESIAN_POINT('Ctrl Pts',(255.37734640349,182.844145577473,249.394812561638));
#27769=UNCERTAINTY_MEASURE_WITH_UNIT(LENGTH_MEASURE(0.01),#27808,
'DISTANCE_ACCURACY_VALUE',
'Maximum model space distance between geometric entities at asserted c
onnectivities');
#27778=UNCERTAINTY_MEASURE_WITH_UNIT(LENGTH_MEASURE(0.01),#27808,
'DISTANCE_ACCURACY_VALUE',
'Maximum model space distance between geometric entities at asserted c
onnectivities');
#27798=(
GEOMETRIC_REPRESENTATION_CONTEXT(3)
GLOBAL_UNCERTAINTY_ASSIGNED_CONTEXT((#27769))
GLOBAL_UNIT_ASSIGNED_CONTEXT((#27808,#27810,#27811))
REPRESENTATION_CONTEXT('','3D')
);
#27807=(
GEOMETRIC_REPRESENTATION_CONTEXT(3)
GLOBAL_UNCERTAINTY_ASSIGNED_CONTEXT((#27778))
GLOBAL_UNIT_ASSIGNED_CONTEXT((#27808,#27810,#27811))
REPRESENTATION_CONTEXT('','3D')
);
#27808=(
LENGTH_UNIT()
NAMED_UNIT(*)
SI_UNIT(.MILLI.,.METRE.)
);
#27810=(
NAMED_UNIT(*)
PLANE_ANGLE_UNIT()
SI_UNIT($,.RADIAN.)
);
#27811=(
NAMED_UNIT(*)
SI_UNIT($,.STERADIAN.)
SOLID_ANGLE_UNIT()
);
#27831=SHAPE_DEFINITION_REPRESENTATION(#27871,#27918);
#27871=PRODUCT_DEFINITION_SHAPE('',$,#27947);
#27918=SHAPE_REPRESENTATION('',(#13369),#27798);
#27927=PRODUCT_DEFINITION_CONTEXT('part definition',#28013,'design');
#27947=PRODUCT_DEFINITION('Handle Socket','Handle Socket',#27975,#27927);
#27975=PRODUCT_DEFINITION_FORMATION('',$,#28034);
#28013=APPLICATION_CONTEXT('Managed model based 3d engineering');
#28014=PRODUCT_CONTEXT('part definition',#28013,'mechanical');
#28034=PRODUCT('Handle Socket','Handle Socket',$,(#28014));
#28064=COLOUR_RGB('Sky Blue',0.24,0.69,0.87);
#28065=FILL_AREA_STYLE_COLOUR('',#28064);
#28066=FILL_AREA_STYLE('',(#28065));
#28067=SURFACE_STYLE_FILL_AREA(#28066);
#28068=SURFACE_SIDE_STYLE('',(#28067));
#28069=SURFACE_STYLE_USAGE(.BOTH.,#28068);
#28070=PRESENTATION_STYLE_ASSIGNMENT((#28069));
ENDSEC;
END-ISO-10303-21;
